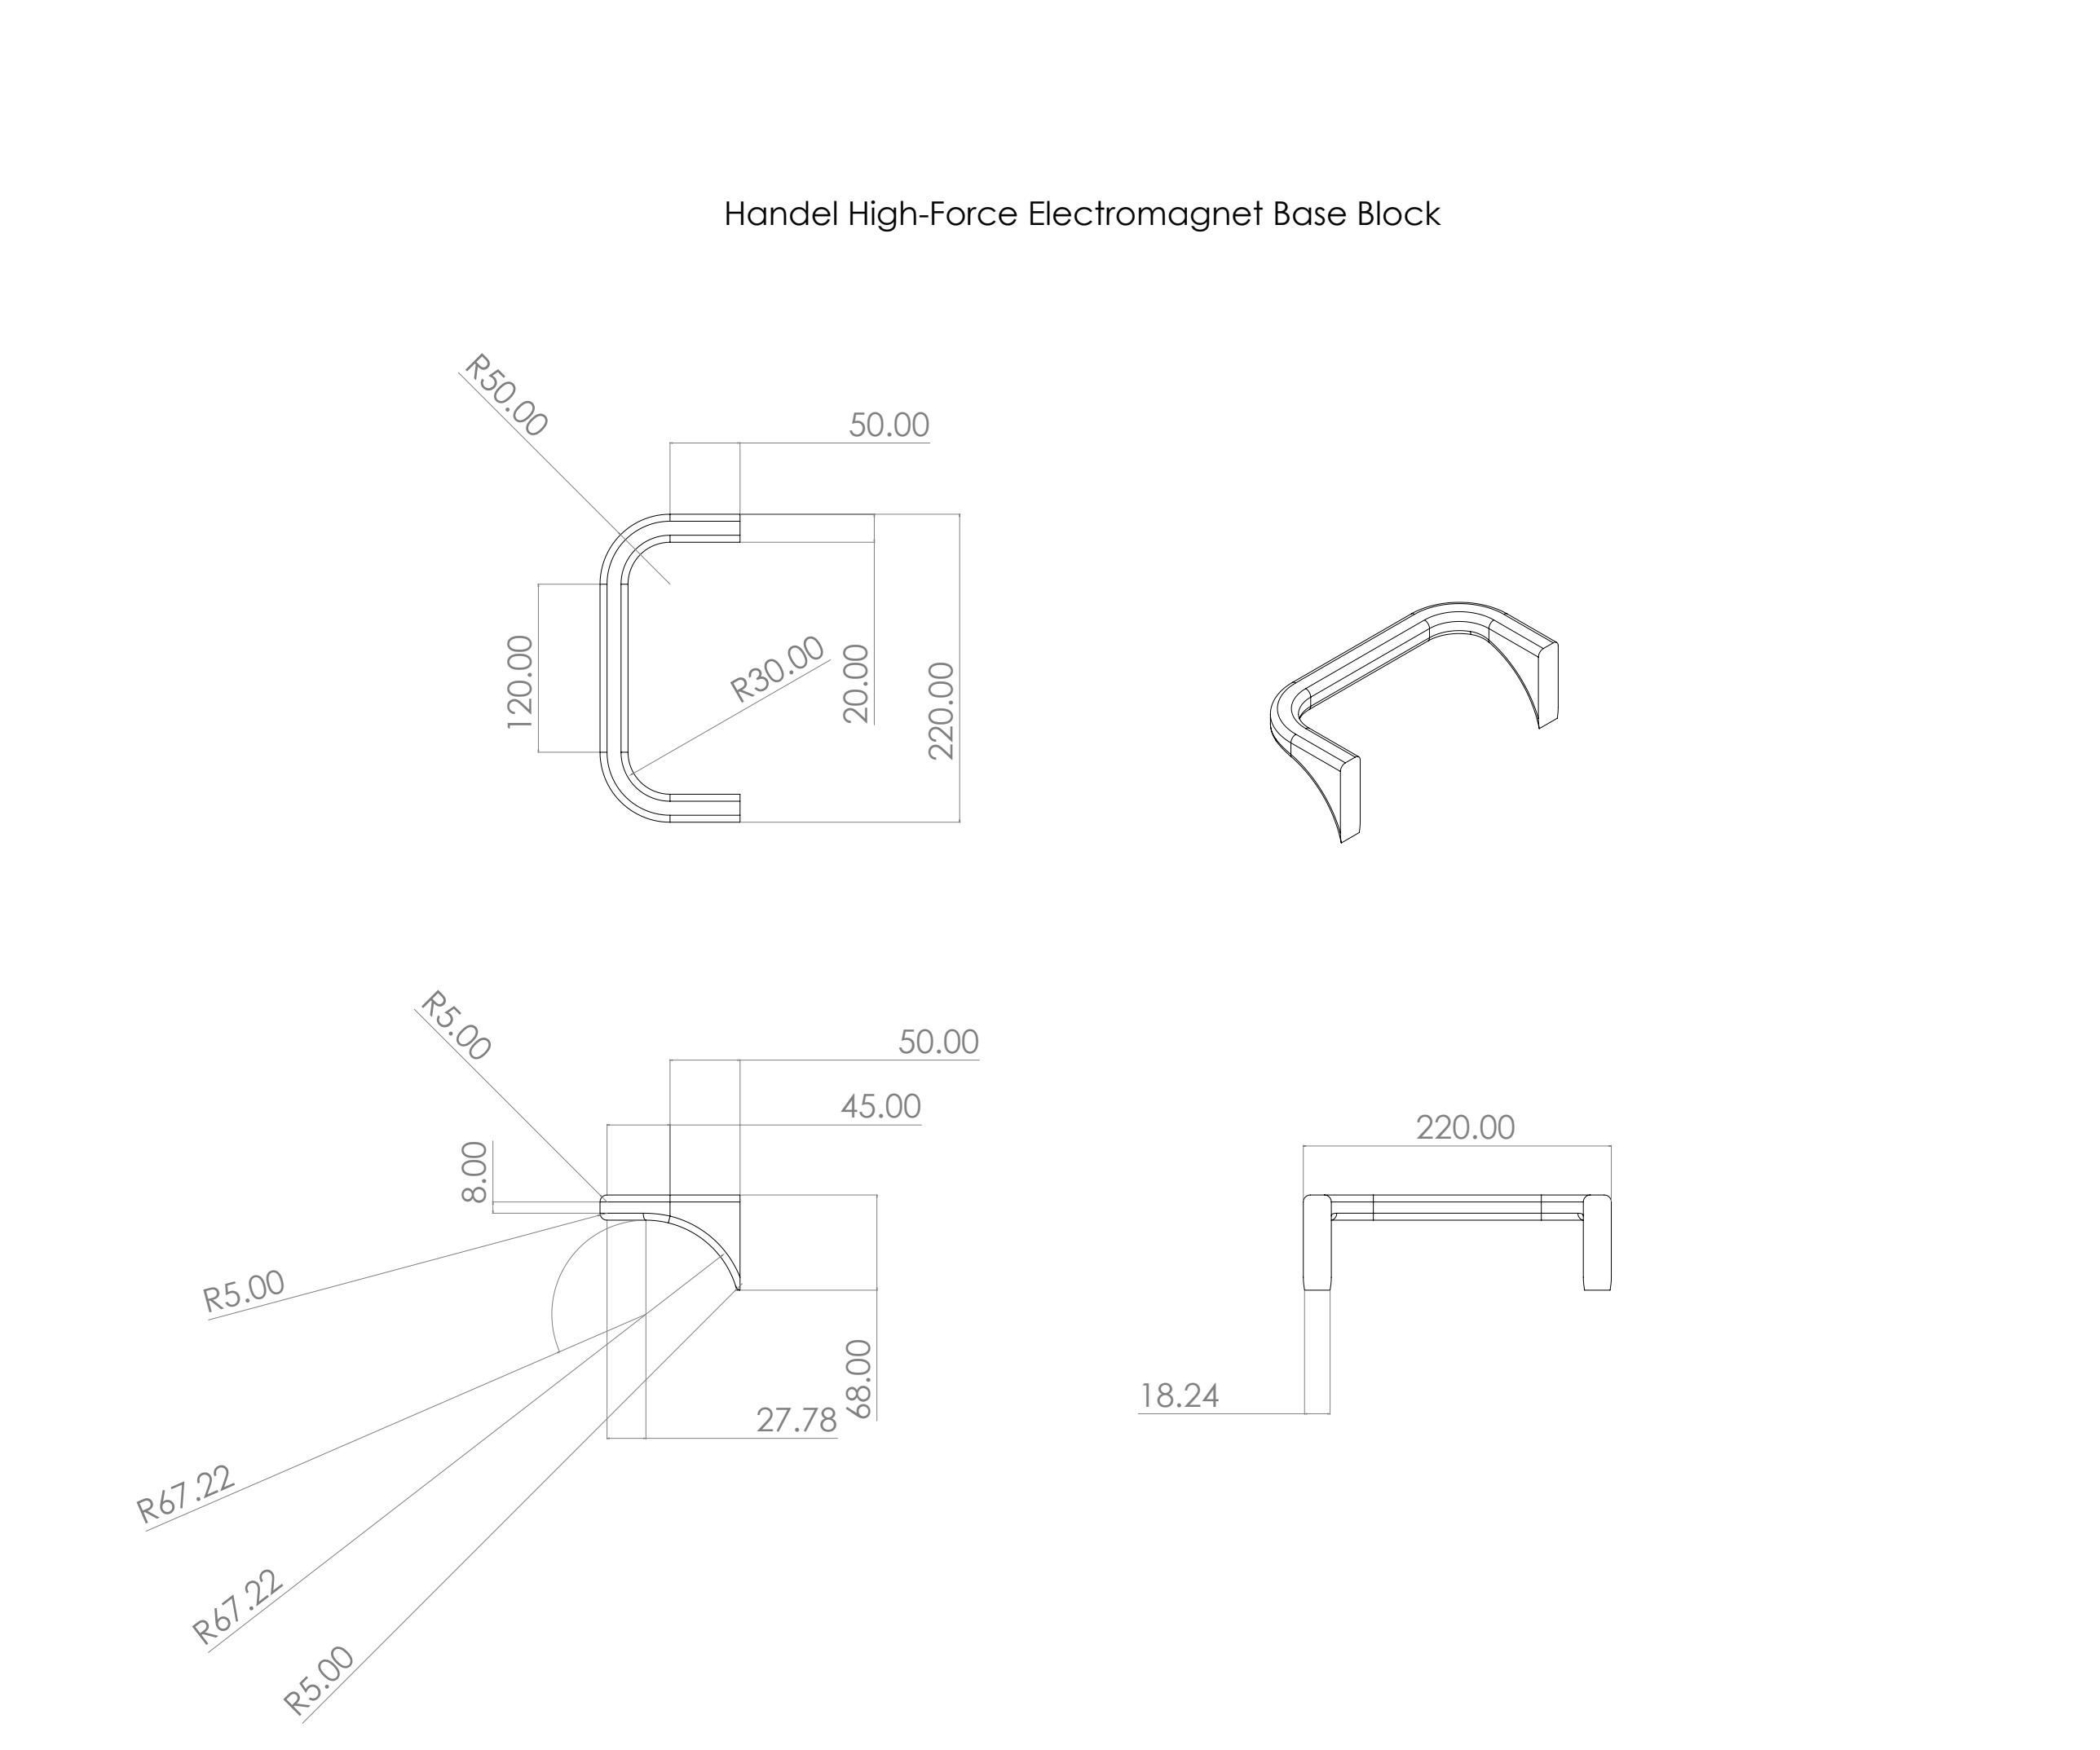
ISO-10303-21;
HEADER;
FILE_DESCRIPTION (('STEP AP214'),
    '1' );
FILE_NAME ('Handel High-Force Electromagnet Base Block.step',
    '2026-10-24T00:09:50',
    ( '' ),
    ( '' ),
    'SwSTEP 2.0',
    'SolidWorks 2025',
    '' );
FILE_SCHEMA (( 'AUTOMOTIVE_DESIGN' ));
ENDSEC;

DATA;
#89=CARTESIAN_POINT ( 'NONE',  ( -260.0000000000001137, -157.0000000000000284, -109.9999999999998721 ) ) ;
#164=CARTESIAN_POINT ( 'NONE',  ( -211.9382648910248861, -218.8137564101509724, 107.3933716542343575 ) ) ;
#173=ADVANCED_FACE ( 'NONE', ( #5707 ), #18920, .T. ) ;
#175=CYLINDRICAL_SURFACE ( 'NONE', #3295, 5.000000000000004441 ) ;
#187=DIRECTION ( 'NONE',  ( 0.000000000000000000, 0.000000000000000000, 1.000000000000000000 ) ) ;
#211=CARTESIAN_POINT ( 'NONE',  ( -260.0000000000001137, -220.0000000000000853, 110.0000000000000142 ) ) ;
#234=EDGE_LOOP ( 'NONE', ( #15831, #2366, #304, #19218 ) ) ;
#245=CARTESIAN_POINT ( 'NONE',  ( -260.0000000000001137, -165.0000000000001137, 60.00000000000002132 ) ) ;
#268=VERTEX_POINT ( 'NONE', #24222 ) ;
#275=VECTOR ( 'NONE', #1072, 1000.000000000000000 ) ;
#288=DIRECTION ( 'NONE',  ( -1.321694076934710155E-16, 1.000000000000000000, 0.000000000000000000 ) ) ;
#301=VERTEX_POINT ( 'NONE', #89 ) ;
#304=ORIENTED_EDGE ( 'NONE', *, *, #26732, .T. ) ;
#312=CARTESIAN_POINT ( 'NONE',  ( -213.1827219047386848, -216.7767438708612531, 105.0000000000000142 ) ) ;
#400=EDGE_CURVE ( 'NONE', #4420, #2951, #20623, .T. ) ;
#420=DIRECTION ( 'NONE',  ( 1.000000000000000000, 0.000000000000000000, 0.000000000000000000 ) ) ;
#473=ADVANCED_FACE ( 'NONE', ( #3894 ), #19413, .T. ) ;
#491=CARTESIAN_POINT ( 'NONE',  ( -270.0517793156885205, -165.1952670567707173, -88.29534001765418338 ) ) ;
#500=ORIENTED_EDGE ( 'NONE', *, *, #25165, .F. ) ;
#515=CARTESIAN_POINT ( 'NONE',  ( -263.9103269956589770, -171.2705086194569901, -104.9999999999999005 ) ) ;
#522=EDGE_LOOP ( 'NONE', ( #13816, #10578, #2122, #14859 ) ) ;
#539=ADVANCED_FACE ( 'NONE', ( #26156 ), #27734, .T. ) ;
#586=CARTESIAN_POINT ( 'NONE',  ( -210.0000000000000568, -157.0000000000000284, -94.99999999999987210 ) ) ;
#591=CARTESIAN_POINT ( 'NONE',  ( -260.0000000000001137, -167.0819201924624906, -109.9999999999998721 ) ) ;
#594=AXIS2_PLACEMENT_3D ( 'NONE', #26284, #2003, #28279 ) ;
#596=ORIENTED_EDGE ( 'NONE', *, *, #20943, .T. ) ;
#618=ORIENTED_EDGE ( 'NONE', *, *, #5223, .T. ) ;
#630=AXIS2_PLACEMENT_3D ( 'NONE', #3020, #873, #5034 ) ;
#631=LINE ( 'NONE', #7377, #27214 ) ;
#681=CARTESIAN_POINT ( 'NONE',  ( -262.5451564304015619, -171.6056065411685552, 105.0000000000519549 ) ) ;
#690=CARTESIAN_POINT ( 'NONE',  ( -210.0000000000000568, -210.8114316696540982, 110.0000000000000284 ) ) ;
#710=VECTOR ( 'NONE', #14587, 1000.000000000000000 ) ;
#721=AXIS2_PLACEMENT_3D ( 'NONE', #25156, #27436, #16685 ) ;
#750=VECTOR ( 'NONE', #15038, 1000.000000000000000 ) ;
#790=ORIENTED_EDGE ( 'NONE', *, *, #25750, .F. ) ;
#802=DIRECTION ( 'NONE',  ( 0.000000000000000000, 1.000000000000000000, 0.000000000000000000 ) ) ;
#817=CARTESIAN_POINT ( 'NONE',  ( -267.9882009536668193, -170.6226266830407496, 104.4279108778009828 ) ) ;
#821=DIRECTION ( 'NONE',  ( -0.8706753206611566043, -1.365180738000214426E-15, -0.4918581970360891842 ) ) ;
#844=CARTESIAN_POINT ( 'NONE',  ( -210.0000000000000000, -218.4793454996983826, 90.61920026979468901 ) ) ;
#865=CARTESIAN_POINT ( 'NONE',  ( -260.0000000000001137, -220.0000000000000853, 90.00000000000001421 ) ) ;
#873=DIRECTION ( 'NONE',  ( 0.9711705445023437466, -0.2383857661250380899, 0.000000000000000000 ) ) ;
#881=DIRECTION ( 'NONE',  ( -1.000000000000000000, 0.000000000000000000, 0.000000000000000000 ) ) ;
#921=DIRECTION ( 'NONE',  ( 4.540956701092242152E-16, 1.000000000000000000, 0.000000000000000000 ) ) ;
#932=CARTESIAN_POINT ( 'NONE',  ( -266.6125751775834942, -170.7865253013266056, -104.7181492081291765 ) ) ;
#973=CARTESIAN_POINT ( 'NONE',  ( -211.6502095576267948, -220.0000000000000568, -92.65159606798890479 ) ) ;
#974=TOROIDAL_SURFACE ( 'NONE', #19304, 44.99999999999999289, 5.000000000000000000 ) ;
#978=CARTESIAN_POINT ( 'NONE',  ( -295.0000000000001137, -170.0000000000001137, 60.00000000000002842 ) ) ;
#984=CARTESIAN_POINT ( 'NONE',  ( -260.0000000000001137, -157.0000000000000284, 60.00000000000002132 ) ) ;
#985=DIRECTION ( 'NONE',  ( -1.000000000000000000, 4.540956701092242152E-16, 0.000000000000000000 ) ) ;
#995=EDGE_LOOP ( 'NONE', ( #6255, #19786, #27111, #10655, #13692 ) ) ;
#1041=CYLINDRICAL_SURFACE ( 'NONE', #20624, 30.00000000000002842 ) ;
#1072=DIRECTION ( 'NONE',  ( -0.000000000000000000, -0.000000000000000000, -1.000000000000000000 ) ) ;
#1181=CARTESIAN_POINT ( 'NONE',  ( -210.0000000000000568, -210.8114316696540982, -89.99999999999987210 ) ) ;
#1212=CARTESIAN_POINT ( 'NONE',  ( -260.0000000000001137, -157.0000000000000284, 90.00000000000001421 ) ) ;
#1263=CARTESIAN_POINT ( 'NONE',  ( -266.7368518929977768, -170.8180696079899121, -94.49756868224339712 ) ) ;
#1264=LINE ( 'NONE', #16233, #14272 ) ;
#1292=LINE ( 'NONE', #27842, #24087 ) ;
#1329=CARTESIAN_POINT ( 'NONE',  ( -295.0000000000002274, -157.0000000000000284, -109.9999999999999858 ) ) ;
#1368=LINE ( 'NONE', #1645, #8748 ) ;
#1386=DIRECTION ( 'NONE',  ( -0.9711705445023439687, 0.2383857661250367854, 0.000000000000000000 ) ) ;
#1401=CARTESIAN_POINT ( 'NONE',  ( -262.3765419278357740, -171.6469950468170111, 89.94932042693801577 ) ) ;
#1411=CARTESIAN_POINT ( 'NONE',  ( -260.0000000000001137, -152.0000000000000284, 60.00000000000002132 ) ) ;
#1429=CARTESIAN_POINT ( 'NONE',  ( -279.1278187736259611, -165.0000000000001137, -106.1966075482097978 ) ) ;
#1432=AXIS2_PLACEMENT_3D ( 'NONE', #1964, #14773, #18933 ) ;
#1459=DIRECTION ( 'NONE',  ( 0.9239321509641974517, 1.061807240666843741E-15, 0.3825563754725196941 ) ) ;
#1468=PLANE ( 'NONE',  #18635 ) ;
#1469=DIRECTION ( 'NONE',  ( -1.321694076934710155E-16, 1.000000000000000000, 0.000000000000000000 ) ) ;
#1495=CARTESIAN_POINT ( 'NONE',  ( -210.0000000000000568, -220.0000000000000853, -109.1217062362807155 ) ) ;
#1508=DIRECTION ( 'NONE',  ( -1.321694076934710155E-16, 1.000000000000000000, 0.000000000000000000 ) ) ;
#1567=EDGE_LOOP ( 'NONE', ( #19464, #20883, #3429, #20222 ) ) ;
#1570=EDGE_CURVE ( 'NONE', #9462, #6741, #17622, .T. ) ;
#1583=TOROIDAL_SURFACE ( 'NONE', #22239, 45.00000000000000711, 5.000000000000000000 ) ;
#1590=EDGE_CURVE ( 'NONE', #16800, #27270, #27778, .T. ) ;
#1603=CIRCLE ( 'NONE', #25453, 5.000000000000004441 ) ;
#1620=EDGE_CURVE ( 'NONE', #28289, #17098, #27637, .T. ) ;
#1645=CARTESIAN_POINT ( 'NONE',  ( -210.0000000000000568, -220.0000000000000853, -89.99999999999987210 ) ) ;
#1655=CARTESIAN_POINT ( 'NONE',  ( -210.0000000000000568, -157.0000000000000284, 90.00000000000002842 ) ) ;
#1659=CYLINDRICAL_SURFACE ( 'NONE', #24420, 5.000000000000004441 ) ;
#1701=ORIENTED_EDGE ( 'NONE', *, *, #1570, .T. ) ;
#1715=CARTESIAN_POINT ( 'NONE',  ( -210.0000000000000568, -157.0000000000000284, 95.00000000000004263 ) ) ;
#1727=AXIS2_PLACEMENT_3D ( 'NONE', #17796, #18378, #985 ) ;
#1732=EDGE_LOOP ( 'NONE', ( #3173, #18800, #24385, #25189 ) ) ;
#1742=CYLINDRICAL_SURFACE ( 'NONE', #24674, 5.000000000000004441 ) ;
#1743=CARTESIAN_POINT ( 'NONE',  ( -260.0000000000001137, -152.0000000000000284, 105.0000000000000142 ) ) ;
#1762=DIRECTION ( 'NONE',  ( -1.321694076934710155E-16, 1.000000000000000000, 0.000000000000000000 ) ) ;
#1792=CARTESIAN_POINT ( 'NONE',  ( -262.5215738956072755, -166.3598102777078509, 89.99999999999998579 ) ) ;
#1810=ADVANCED_FACE ( 'NONE', ( #6661 ), #11116, .T. ) ;
#1812=PLANE ( 'NONE',  #12527 ) ;
#1817=CARTESIAN_POINT ( 'NONE',  ( -267.0129679999498649, -170.7675089197775264, -89.18277029719632765 ) ) ;
#1818=CARTESIAN_POINT ( 'NONE',  ( -266.3037744482016365, -165.6613878827935196, 89.35851331749265114 ) ) ;
#1821=CARTESIAN_POINT ( 'NONE',  ( -262.5802634612744555, -171.5969890882419406, -94.99999999999990052 ) ) ;
#1833=VECTOR ( 'NONE', #27757, 1000.000000000000000 ) ;
#1849=CARTESIAN_POINT ( 'NONE',  ( -271.2644327268766915, -165.3329768350718041, -108.7419004184296369 ) ) ;
#1882=EDGE_CURVE ( 'NONE', #21087, #5617, #8959, .T. ) ;
#1937=DIRECTION ( 'NONE',  ( 0.000000000000000000, 0.000000000000000000, -1.000000000000000000 ) ) ;
#1957=CARTESIAN_POINT ( 'NONE',  ( -266.0153270024459289, -170.9359483083451039, -94.62226971369513251 ) ) ;
#1958=CARTESIAN_POINT ( 'NONE',  ( -270.3796563303090466, -170.3242331377992684, 88.15587544550923838 ) ) ;
#1964=CARTESIAN_POINT ( 'NONE',  ( -277.2150368962633706, -237.2150368962634559, -109.9999999999998153 ) ) ;
#1993=ADVANCED_FACE ( 'NONE', ( #20301 ), #18155, .F. ) ;
#2002=CARTESIAN_POINT ( 'NONE',  ( -210.0000000000000568, -220.0000000000000853, 110.0000000000000284 ) ) ;
#2003=DIRECTION ( 'NONE',  ( -4.540956701092242152E-16, -1.000000000000000000, -0.000000000000000000 ) ) ;
#2019=EDGE_CURVE ( 'NONE', #17098, #12396, #27748, .T. ) ;
#2064=CARTESIAN_POINT ( 'NONE',  ( -262.5514013678064771, -171.6040736444017512, 105.0000000000000000 ) ) ;
#2073=ORIENTED_EDGE ( 'NONE', *, *, #6135, .T. ) ;
#2074=LINE ( 'NONE', #13160, #28386 ) ;
#2091=ORIENTED_EDGE ( 'NONE', *, *, #5972, .T. ) ;
#2096=CARTESIAN_POINT ( 'NONE',  ( -213.1248215185737820, -216.9499264940854744, 94.81074245358750829 ) ) ;
#2104=DIRECTION ( 'NONE',  ( -0.000000000000000000, -1.000000000000000000, -0.000000000000000000 ) ) ;
#2122=ORIENTED_EDGE ( 'NONE', *, *, #1590, .T. ) ;
#2143=DIRECTION ( 'NONE',  ( -1.000000000000000000, -9.204883169708156517E-49, 3.053113317719176542E-15 ) ) ;
#2151=SHAPE_DEFINITION_REPRESENTATION ( #25856, #3128 ) ;
#2258=AXIS2_PLACEMENT_3D ( 'NONE', #11059, #12938, #28277 ) ;
#2296=AXIS2_PLACEMENT_3D ( 'NONE', #27206, #12280, #10255 ) ;
#2320=DIRECTION ( 'NONE',  ( 0.000000000000000000, 0.000000000000000000, 1.000000000000000000 ) ) ;
#2351=CIRCLE ( 'NONE', #1432, 72.21503689626329958 ) ;
#2364=ORIENTED_EDGE ( 'NONE', *, *, #6001, .T. ) ;
#2366=ORIENTED_EDGE ( 'NONE', *, *, #15464, .T. ) ;
#2410=AXIS2_PLACEMENT_3D ( 'NONE', #19417, #16704, #20998 ) ;
#2419=CARTESIAN_POINT ( 'NONE',  ( -310.0000000000001137, -220.0000000000000853, -59.99999999999987210 ) ) ;
#2453=ADVANCED_FACE ( 'NONE', ( #8296 ), #5320, .T. ) ;
#2463=EDGE_LOOP ( 'NONE', ( #27973, #3663, #26251, #20729 ) ) ;
#2472=EDGE_CURVE ( 'NONE', #9488, #19744, #24227, .T. ) ;
#2494=ADVANCED_FACE ( 'NONE', ( #19915 ), #25006, .T. ) ;
#2502=DIRECTION ( 'NONE',  ( -1.321694076934710155E-16, 1.000000000000000000, 0.000000000000000000 ) ) ;
#2527=EDGE_CURVE ( 'NONE', #9488, #23090, #13611, .T. ) ;
#2532=LINE ( 'NONE', #22518, #11233 ) ;
#2542=ORIENTED_EDGE ( 'NONE', *, *, #24570, .T. ) ;
#2556=DIRECTION ( 'NONE',  ( -0.000000000000000000, -0.000000000000000000, 1.000000000000000000 ) ) ;
#2566=ADVANCED_FACE ( 'NONE', ( #24094 ), #8859, .T. ) ;
#2593=CARTESIAN_POINT ( 'NONE',  ( -213.1248215185737820, -216.9499264940855028, 105.1892575464125770 ) ) ;
#2608=DIRECTION ( 'NONE',  ( -1.000000000000000000, -0.000000000000000000, 2.775557561562887407E-16 ) ) ;
#2621=DIRECTION ( 'NONE',  ( -0.000000000000000000, -1.000000000000000000, -0.000000000000000000 ) ) ;
#2625=CARTESIAN_POINT ( 'NONE',  ( -260.0000000000001137, -170.0000000000001137, 60.00000000000002132 ) ) ;
#2634=ADVANCED_FACE ( 'NONE', ( #26951 ), #22652, .T. ) ;
#2676=CARTESIAN_POINT ( 'NONE',  ( -277.2150368962633706, -237.2150368962634559, 95.00000000000004263 ) ) ;
#2686=ORIENTED_EDGE ( 'NONE', *, *, #1570, .F. ) ;
#2687=DIRECTION ( 'NONE',  ( -0.000000000000000000, -0.000000000000000000, -1.000000000000000000 ) ) ;
#2715=STYLED_ITEM('',(#28420),#27732);
#2771=DIRECTION ( 'NONE',  ( 4.540956701092242152E-16, 1.000000000000000000, 0.000000000000000000 ) ) ;
#2777=CARTESIAN_POINT ( 'NONE',  ( -290.0000000000001137, -157.0000000000000284, 60.00000000000002842 ) ) ;
#2785=ORIENTED_EDGE ( 'NONE', *, *, #10230, .T. ) ;
#2798=CARTESIAN_POINT ( 'NONE',  ( -261.1919288306253293, -171.9377729149742038, -104.9999999999998721 ) ) ;
#2815=CARTESIAN_POINT ( 'NONE',  ( -272.9143904460767658, -165.1584295805091642, 108.4134862853730965 ) ) ;
#2830=B_SPLINE_CURVE_WITH_KNOTS ( 'NONE', 3,
 ( #15606, #24348, #4662, #13445, #19754, #4381, #12886, #22201, #19618, #26357, #24215, #23935 ),
 .UNSPECIFIED., .F., .F.,
 ( 4, 2, 2, 2, 2, 4 ),
 ( 0.000000000000000000, 0.004258726182425120153, 0.006388089273637603469, 0.008517452364850087651, 0.01277617854727505428, 0.01703490472970001918 ),
 .UNSPECIFIED. ) ;
#2857=CIRCLE ( 'NONE', #5602, 5.000000000000004441 ) ;
#2934=EDGE_CURVE ( 'NONE', #6860, #23545, #18607, .T. ) ;
#2945=CARTESIAN_POINT ( 'NONE',  ( -277.2150368962633706, -170.0000000000001137, 101.5769467933889558 ) ) ;
#2951=VERTEX_POINT ( 'NONE', #24194 ) ;
#2963=CARTESIAN_POINT ( 'NONE',  ( -261.1919288306253293, -171.9377729149742038, 105.0000000000000142 ) ) ;
#2972=DIRECTION ( 'NONE',  ( -1.321694076934710155E-16, 1.000000000000000000, 0.000000000000000000 ) ) ;
#2992=AXIS2_PLACEMENT_3D ( 'NONE', #7090, #26770, #20999 ) ;
#3020=CARTESIAN_POINT ( 'NONE',  ( -260.0000000000001137, -167.0819201924624906, 105.0000000000000142 ) ) ;
#3073=VECTOR ( 'NONE', #26874, 1000.000000000000000 ) ;
#3078=ORIENTED_EDGE ( 'NONE', *, *, #1620, .F. ) ;
#3095=CARTESIAN_POINT ( 'NONE',  ( -268.7660490202469532, -170.5116556248577524, 109.2537565056162379 ) ) ;
#3103=AXIS2_PLACEMENT_3D ( 'NONE', #28274, #8473, #17230 ) ;
#3128=SHAPE_REPRESENTATION ( 'Handel High-Force Electromagnet Base Block', ( #10637 ), #6979 ) ;
#3142=AXIS2_PLACEMENT_3D ( 'NONE', #11715, #22040, #15736 ) ;
#3144=DIRECTION ( 'NONE',  ( 0.000000000000000000, 0.000000000000000000, 1.000000000000000000 ) ) ;
#3147=VERTEX_POINT ( 'NONE', #2777 ) ;
#3173=ORIENTED_EDGE ( 'NONE', *, *, #15521, .T. ) ;
#3224=VERTEX_POINT ( 'NONE', #591 ) ;
#3236=CARTESIAN_POINT ( 'NONE',  ( -264.2078319525319898, -171.2518620402580325, 109.8556748947001296 ) ) ;
#3248=CARTESIAN_POINT ( 'NONE',  ( -260.0000000000001137, -167.0819201924624906, -94.99999999999987210 ) ) ;
#3272=DIRECTION ( 'NONE',  ( 0.3825563754725206378, 0.000000000000000000, 0.9239321509641971186 ) ) ;
#3295=AXIS2_PLACEMENT_3D ( 'NONE', #22146, #26589, #17410 ) ;
#3306=FACE_OUTER_BOUND ( 'NONE', #14305, .T. ) ;
#3316=PRODUCT_DEFINITION ( 'UNKNOWN', '', #4206, #7165 ) ;
#3325=CARTESIAN_POINT ( 'NONE',  ( -212.2419371577844345, -220.0000000000000853, -105.0000000000000284 ) ) ;
#3345=AXIS2_PLACEMENT_3D ( 'NONE', #5821, #12027, #12311 ) ;
#3349=AXIS2_PLACEMENT_3D ( 'NONE', #25379, #1386, #5699 ) ;
#3353=PLANE ( 'NONE',  #2296 ) ;
#3368=VERTEX_POINT ( 'NONE', #9476 ) ;
#3407=EDGE_CURVE ( 'NONE', #3147, #8779, #22883, .T. ) ;
#3418=CARTESIAN_POINT ( 'NONE',  ( -277.2150368962633706, -170.0000000000001137, -90.47363622314027509 ) ) ;
#3428=AXIS2_PLACEMENT_3D ( 'NONE', #27338, #9833, #11858 ) ;
#3429=ORIENTED_EDGE ( 'NONE', *, *, #9744, .F. ) ;
#3430=ORIENTED_EDGE ( 'NONE', *, *, #16149, .T. ) ;
#3448=FACE_OUTER_BOUND ( 'NONE', #16029, .T. ) ;
#3451=EDGE_CURVE ( 'NONE', #18918, #10091, #26206, .T. ) ;
#3457=CIRCLE ( 'NONE', #12242, 29.99999999999997158 ) ;
#3491=DIRECTION ( 'NONE',  ( -0.000000000000000000, -0.000000000000000000, 1.000000000000000000 ) ) ;
#3513=CARTESIAN_POINT ( 'NONE',  ( -210.0000000000000568, -216.9546086794800317, 109.5971846486504404 ) ) ;
#3520=DIRECTION ( 'NONE',  ( 1.000000000000000000, 0.000000000000000000, 2.775557561562887407E-16 ) ) ;
#3529=DIRECTION ( 'NONE',  ( 0.2383857661250380344, 0.9711705445023436356, 0.000000000000000000 ) ) ;
#3545=CARTESIAN_POINT ( 'NONE',  ( -277.2150368962633706, -170.0000000000001137, -90.47363622314027509 ) ) ;
#3547=CARTESIAN_POINT ( 'NONE',  ( -269.2495632547581863, -170.4544034111251278, 88.54864639839837537 ) ) ;
#3567=ORIENTED_EDGE ( 'NONE', *, *, #2527, .F. ) ;
#3577=CARTESIAN_POINT ( 'NONE',  ( -260.0000000000001137, -220.0000000000000853, 60.00000000000002132 ) ) ;
#3590=AXIS2_PLACEMENT_3D ( 'NONE', #15942, #20233, #420 ) ;
#3591=CARTESIAN_POINT ( 'NONE',  ( -266.4480630393687193, -165.8483660650564389, -109.6897131948989568 ) ) ;
#3602=CARTESIAN_POINT ( 'NONE',  ( -210.0000000000000568, -152.0000000000000284, -110.0000000000000284 ) ) ;
#3641=CARTESIAN_POINT ( 'NONE',  ( -210.0000000000000568, -210.8114316696540982, 90.00000000000002842 ) ) ;
#3663=ORIENTED_EDGE ( 'NONE', *, *, #5671, .F. ) ;
#3686=CARTESIAN_POINT ( 'NONE',  ( -266.9759726783797191, -165.5689182401532946, -89.18477089400076352 ) ) ;
#3699=DIRECTION ( 'NONE',  ( 0.000000000000000000, 0.000000000000000000, -1.000000000000000000 ) ) ;
#3702=VERTEX_POINT ( 'NONE', #14768 ) ;
#3720=CARTESIAN_POINT ( 'NONE',  ( -277.5942566850414437, -165.0000000000001705, -106.8315826960697450 ) ) ;
#3746=DIRECTION ( 'NONE',  ( -0.000000000000000000, -0.000000000000000000, 1.000000000000000000 ) ) ;
#3780=ORIENTED_EDGE ( 'NONE', *, *, #13513, .F. ) ;
#3781=AXIS2_PLACEMENT_3D ( 'NONE', #27138, #24992, #22976 ) ;
#3845=ORIENTED_EDGE ( 'NONE', *, *, #13749, .F. ) ;
#3873=LINE ( 'NONE', #12662, #17378 ) ;
#3884=ORIENTED_EDGE ( 'NONE', *, *, #1882, .F. ) ;
#3894=FACE_OUTER_BOUND ( 'NONE', #522, .T. ) ;
#3931=ADVANCED_FACE ( 'NONE', ( #21289 ), #14556, .T. ) ;
#3950=CARTESIAN_POINT ( 'NONE',  ( -260.0000000000001137, -167.0819201924624906, 90.00000000000001421 ) ) ;
#3969=DIRECTION ( 'NONE',  ( 1.321694076934710155E-16, -1.000000000000000000, 0.000000000000000000 ) ) ;
#3972=CARTESIAN_POINT ( 'NONE',  ( -268.8456629416622263, -165.3150191422601551, -88.69519881272435669 ) ) ;
#3973=CARTESIAN_POINT ( 'NONE',  ( -263.9427288773140390, -171.3087732700370225, 94.90640018636418063 ) ) ;
#3995=ADVANCED_FACE ( 'NONE', ( #12268 ), #1742, .T. ) ;
#4005=CARTESIAN_POINT ( 'NONE',  ( -305.0000000000001137, -165.0000000000000853, -59.99999999999987210 ) ) ;
#4017=CARTESIAN_POINT ( 'NONE',  ( -271.2500882473517549, -165.3342412936102050, -108.7452232840771558 ) ) ;
#4093=LINE ( 'NONE', #10997, #7349 ) ;
#4102=ORIENTED_EDGE ( 'NONE', *, *, #25165, .T. ) ;
#4115=CARTESIAN_POINT ( 'NONE',  ( -262.5702831125496459, -171.5994388877033998, -94.99999999999987210 ) ) ;
#4138=ORIENTED_EDGE ( 'NONE', *, *, #22755, .T. ) ;
#4161=CARTESIAN_POINT ( 'NONE',  ( -270.6159714707433182, -170.3110992094025278, -103.8707009556082994 ) ) ;
#4206=PRODUCT_DEFINITION_FORMATION_WITH_SPECIFIED_SOURCE ( 'ANY', '', #4537, .NOT_KNOWN. ) ;
#4251=VERTEX_POINT ( 'NONE', #14381 ) ;
#4255=CARTESIAN_POINT ( 'NONE',  ( -210.4359063544880541, -219.8547609215023328, 91.14353391724667119 ) ) ;
#4261=CARTESIAN_POINT ( 'NONE',  ( -210.0000000000000568, -152.0000000000000284, -110.0000000000000284 ) ) ;
#4264=CARTESIAN_POINT ( 'NONE',  ( -260.0000000000001137, -152.0000000000000284, -59.99999999999986500 ) ) ;
#4284=EDGE_LOOP ( 'NONE', ( #500, #10010, #26500, #14827 ) ) ;
#4381=CARTESIAN_POINT ( 'NONE',  ( -270.7820719900048516, -170.3051706208958365, 93.45761744549247396 ) ) ;
#4420=VERTEX_POINT ( 'NONE', #15232 ) ;
#4447=ORIENTED_EDGE ( 'NONE', *, *, #16149, .F. ) ;
#4503=ADVANCED_FACE ( 'NONE', ( #28133 ), #8757, .F. ) ;
#4519=CARTESIAN_POINT ( 'NONE',  ( -268.1249842685929821, -165.6674762674429076, 109.3623863443581570 ) ) ;
#4528=AXIS2_PLACEMENT_3D ( 'NONE', #22625, #921, #27062 ) ;
#4537=PRODUCT ( 'Handel High-Force Electromagnet Base Block', 'Handel High-Force Electromagnet Base Block', '', ( #21552 ) ) ;
#4544=FACE_OUTER_BOUND ( 'NONE', #11580, .T. ) ;
#4546=ADVANCED_FACE ( 'NONE', ( #13650 ), #25572, .T. ) ;
#4582=ORIENTED_EDGE ( 'NONE', *, *, #16178, .F. ) ;
#4593=ORIENTED_EDGE ( 'NONE', *, *, #25750, .T. ) ;
#4594=ADVANCED_FACE ( 'NONE', ( #11646 ), #26496, .T. ) ;
#4608=CARTESIAN_POINT ( 'NONE',  ( -210.0000000000000568, -220.0000000000000853, -89.99999999999987210 ) ) ;
#4611=CARTESIAN_POINT ( 'NONE',  ( -211.0655007229363207, -220.0000000000000568, -108.1818347287491378 ) ) ;
#4654=CARTESIAN_POINT ( 'NONE',  ( -295.0000000000001705, -152.0000000000000284, 60.00000000000002842 ) ) ;
#4658=CIRCLE ( 'NONE', #6486, 35.00000000000002842 ) ;
#4662=CARTESIAN_POINT ( 'NONE',  ( -274.7321073701114642, -170.0332518446063830, 91.86918944433702450 ) ) ;
#4680=CARTESIAN_POINT ( 'NONE',  ( -277.2150368962633706, -170.0000000000001137, -90.47363622314027509 ) ) ;
#4739=CARTESIAN_POINT ( 'NONE',  ( -295.0000000000001705, -165.0000000000001137, -59.99999999999986500 ) ) ;
#4757=DIRECTION ( 'NONE',  ( 1.000000000000000000, 0.000000000000000000, -2.775557561562887407E-16 ) ) ;
#4787=EDGE_LOOP ( 'NONE', ( #10218, #10585, #21921, #10657 ) ) ;
#4802=DIRECTION ( 'NONE',  ( 0.000000000000000000, 0.000000000000000000, -1.000000000000000000 ) ) ;
#4823=DIRECTION ( 'NONE',  ( -1.000000000000000000, 0.000000000000000000, 0.000000000000000000 ) ) ;
#4852=UNCERTAINTY_MEASURE_WITH_UNIT (LENGTH_MEASURE( 1.000000000000000082E-05 ), #24383, 'distance_accuracy_value', 'NONE');
#5022=ORIENTED_EDGE ( 'NONE', *, *, #5982, .T. ) ;
#5032=EDGE_CURVE ( 'NONE', #5806, #16800, #18347, .T. ) ;
#5034=DIRECTION ( 'NONE',  ( 0.2383857661250380344, 0.9711705445023436356, 0.000000000000000000 ) ) ;
#5051=ORIENTED_EDGE ( 'NONE', *, *, #6001, .F. ) ;
#5074=CARTESIAN_POINT ( 'NONE',  ( -262.5249090614869374, -166.4079007703013247, -89.92078834904907580 ) ) ;
#5116=CARTESIAN_POINT ( 'NONE',  ( -279.1278187736259611, -170.0000000000001421, 106.1966075482099683 ) ) ;
#5132=ORIENTED_EDGE ( 'NONE', *, *, #28205, .F. ) ;
#5146=EDGE_CURVE ( 'NONE', #16800, #12640, #24714, .T. ) ;
#5157=AXIS2_PLACEMENT_3D ( 'NONE', #15697, #10951, #13397 ) ;
#5223=EDGE_CURVE ( 'NONE', #18214, #19744, #5687, .T. ) ;
#5257=DIRECTION ( 'NONE',  ( -1.000000000000000000, 0.000000000000000000, -0.000000000000000000 ) ) ;
#5279=ORIENTED_EDGE ( 'NONE', *, *, #10174, .T. ) ;
#5295=DIRECTION ( 'NONE',  ( -0.000000000000000000, -0.000000000000000000, 1.000000000000000000 ) ) ;
#5305=ORIENTED_EDGE ( 'NONE', *, *, #22027, .F. ) ;
#5320=( BOUNDED_SURFACE ( )  B_SPLINE_SURFACE ( 3, 2, ( 
 ( #25811, #14913, #28097 ),
 ( #5714, #1401, #23667 ),
 ( #3973, #12760, #6276 ),
 ( #21500, #15050, #19495 ),
 ( #17332, #12340, #1818 ),
 ( #10173, #10592, #28239 ),
 ( #19348, #3547, #12901 ),
 ( #21648, #1958, #14488 ),
 ( #23245, #16779, #18930 ),
 ( #27673, #8013, #13463 ),
 ( #11459, #15195, #15482 ),
 ( #9003, #23952, #22072 ) ),
 .UNSPECIFIED., .F., .F., .F. ) 
 B_SPLINE_SURFACE_WITH_KNOTS ( ( 4, 2, 2, 2, 2, 4 ),
 ( 3, 3 ),
 ( 0.000000000000000000, 0.004509302159734392135, 0.009018604319468784269, 0.01127325539933598034, 0.01352790647920317640, 0.01803720863893756854 ),
 ( 0.000000000000000000, 1.000000000000000000 ),
 .UNSPECIFIED. ) 
 GEOMETRIC_REPRESENTATION_ITEM ( )  RATIONAL_B_SPLINE_SURFACE ( (
 ( 1.000000000000000000, 0.7071067811865475727, 1.000000000000000000),
 ( 1.000000000000000000, 0.7035406144708270526, 1.000000000000000000),
 ( 1.000000000000000000, 0.7008848705186870864, 1.000000000000000000),
 ( 1.000000000000000000, 0.6974083274405008526, 1.000000000000000000),
 ( 1.000000000000000000, 0.6965884901777600335, 1.000000000000000000),
 ( 1.000000000000000000, 0.6967133934288484154, 1.000000000000000000),
 ( 1.000000000000000000, 0.6969819717335956621, 1.000000000000000000),
 ( 1.000000000000000000, 0.6979534373899805022, 1.000000000000000000),
 ( 1.000000000000000000, 0.6986531993633946502, 1.000000000000000000),
 ( 1.000000000000000000, 0.7013382012354564266, 1.000000000000000000),
 ( 1.000000000000000000, 0.7039093929050953546, 1.000000000000000000),
 ( 1.000000000000000000, 0.7071067811865475727, 1.000000000000000000) ) ) 
 REPRESENTATION_ITEM ( '' )  SURFACE ( )  );
#5365=LINE ( 'NONE', #13723, #16606 ) ;
#5377=AXIS2_PLACEMENT_3D ( 'NONE', #3602, #5484, #20857 ) ;
#5382=ORIENTED_EDGE ( 'NONE', *, *, #12688, .F. ) ;
#5387=CARTESIAN_POINT ( 'NONE',  ( -212.2419371577844345, -220.0000000000000853, -94.99999999999987210 ) ) ;
#5477=EDGE_CURVE ( 'NONE', #10903, #10018, #16476, .T. ) ;
#5484=DIRECTION ( 'NONE',  ( 0.000000000000000000, -1.000000000000000000, -0.000000000000000000 ) ) ;
#5499=CARTESIAN_POINT ( 'NONE',  ( -272.4438906011233712, -165.0368527442270477, -87.32790004433633158 ) ) ;
#5507=ORIENTED_EDGE ( 'NONE', *, *, #1882, .T. ) ;
#5526=CARTESIAN_POINT ( 'NONE',  ( -210.0000000000000568, -210.8114316696540982, -110.0000000000000284 ) ) ;
#5534=CARTESIAN_POINT ( 'NONE',  ( -210.0000000000000000, -212.3568517473289035, 110.0000000000000000 ) ) ;
#5541=CARTESIAN_POINT ( 'NONE',  ( -267.2505360800719814, -170.7220645054522663, 109.5009084174815541 ) ) ;
#5553=FACE_OUTER_BOUND ( 'NONE', #10103, .T. ) ;
#5554=VERTEX_POINT ( 'NONE', #21544 ) ;
#5555=CARTESIAN_POINT ( 'NONE',  ( -279.1278187736259611, -165.0000000000001137, -106.1966075482097978 ) ) ;
#5564=CARTESIAN_POINT ( 'NONE',  ( -290.0000000000001705, -157.0000000000000284, -59.99999999999986500 ) ) ;
#5602=AXIS2_PLACEMENT_3D ( 'NONE', #20556, #7498, #881 ) ;
#5617=VERTEX_POINT ( 'NONE', #7393 ) ;
#5662=ORIENTED_EDGE ( 'NONE', *, *, #5477, .T. ) ;
#5669=CARTESIAN_POINT ( 'NONE',  ( -210.0000000000000853, -216.9546086794800601, -109.5971846486504830 ) ) ;
#5671=EDGE_CURVE ( 'NONE', #23545, #15321, #3873, .T. ) ;
#5687=LINE ( 'NONE', #23213, #11873 ) ;
#5699=DIRECTION ( 'NONE',  ( -0.2383857661250380344, -0.9711705445023436356, 0.000000000000000000 ) ) ;
#5707=FACE_OUTER_BOUND ( 'NONE', #995, .T. ) ;
#5712=CARTESIAN_POINT ( 'NONE',  ( -266.7040755562055097, -170.8232809441065001, -94.50355751542548433 ) ) ;
#5714=CARTESIAN_POINT ( 'NONE',  ( -262.5700334248197123, -171.5995001766305847, 94.99999999990480148 ) ) ;
#5723=ORIENTED_EDGE ( 'NONE', *, *, #19780, .F. ) ;
#5728=ORIENTED_EDGE ( 'NONE', *, *, #27879, .T. ) ;
#5748=EDGE_CURVE ( 'NONE', #22565, #22186, #7330, .T. ) ;
#5775=ADVANCED_FACE ( 'NONE', ( #10778 ), #23374, .T. ) ;
#5798=ORIENTED_EDGE ( 'NONE', *, *, #25915, .T. ) ;
#5806=VERTEX_POINT ( 'NONE', #27132 ) ;
#5820=CARTESIAN_POINT ( 'NONE',  ( -260.0000000000001137, -165.0000000000001137, -59.99999999999986500 ) ) ;
#5821=CARTESIAN_POINT ( 'NONE',  ( -310.0000000000001137, -220.0000000000000853, -59.99999999999987210 ) ) ;
#5832=DIRECTION ( 'NONE',  ( -1.000000000000000000, 0.000000000000000000, 0.000000000000000000 ) ) ;
#5842=VERTEX_POINT ( 'NONE', #26990 ) ;
#5847=CARTESIAN_POINT ( 'NONE',  ( -212.1902656986470390, -220.0000000000000284, -94.18570773969327092 ) ) ;
#5849=CARTESIAN_POINT ( 'NONE',  ( -273.6179505379467400, -164.9999999998308624, -86.76301814019983283 ) ) ;
#5875=B_SPLINE_CURVE_WITH_KNOTS ( 'NONE', 3,
 ( #3950, #1792, #10569, #19325, #15317, #26349, #15028, #23780, #17449, #21621 ),
 .UNSPECIFIED., .F., .F.,
 ( 4, 2, 2, 2, 4 ),
 ( 0.000000000000000000, 0.007751866621267358357, 0.009689833276584160215, 0.01162779993190096207, 0.01550373324253456232 ),
 .UNSPECIFIED. ) ;
#5881=DIRECTION ( 'NONE',  ( 0.000000000000000000, 0.000000000000000000, 1.000000000000000000 ) ) ;
#5894=CARTESIAN_POINT ( 'NONE',  ( -271.9547679543769618, -170.1928761609053993, -103.5145866598865183 ) ) ;
#5936=CARTESIAN_POINT ( 'NONE',  ( -295.0000000000002274, -152.0000000000000284, -59.99999999999986500 ) ) ;
#5937=AXIS2_PLACEMENT_3D ( 'NONE', #20996, #1459, #10234 ) ;
#5969=DIRECTION ( 'NONE',  ( -2.775557561562887407E-16, -3.668437989309015850E-32, 1.000000000000000000 ) ) ;
#5971=ORIENTED_EDGE ( 'NONE', *, *, #20762, .T. ) ;
#5972=EDGE_CURVE ( 'NONE', #6357, #18214, #20609, .T. ) ;
#5982=EDGE_CURVE ( 'NONE', #24757, #12396, #14205, .T. ) ;
#5990=CARTESIAN_POINT ( 'NONE',  ( -262.3767685073270286, -171.6469394300385432, -89.94931073348448081 ) ) ;
#6001=EDGE_CURVE ( 'NONE', #21738, #15321, #6003, .T. ) ;
#6002=TOROIDAL_SURFACE ( 'NONE', #16113, 72.21503689626331379, 5.000000000000000000 ) ;
#6003=LINE ( 'NONE', #10181, #17854 ) ;
#6039=CARTESIAN_POINT ( 'NONE',  ( -273.2081292221210447, -170.0913695707084514, -108.2505382271841086 ) ) ;
#6070=VERTEX_POINT ( 'NONE', #3418 ) ;
#6077=CARTESIAN_POINT ( 'NONE',  ( -295.0000000000001705, -170.0000000000001137, -59.99999999999986500 ) ) ;
#6114=DIRECTION ( 'NONE',  ( -1.321694076934710155E-16, 1.000000000000000000, 0.000000000000000000 ) ) ;
#6115=DIRECTION ( 'NONE',  ( -1.000000000000000000, 4.540956701092242152E-16, 0.000000000000000000 ) ) ;
#6116=LINE ( 'NONE', #14746, #23778 ) ;
#6132=CARTESIAN_POINT ( 'NONE',  ( -211.4917091876254744, -219.2061850725015120, 92.08741365143876578 ) ) ;
#6135=EDGE_CURVE ( 'NONE', #12640, #6070, #12377, .T. ) ;
#6136=CARTESIAN_POINT ( 'NONE',  ( -274.7557459110828972, -170.0000000000001137, -86.12025961983449918 ) ) ;
#6175=DIRECTION ( 'NONE',  ( 1.000000000000000000, 0.000000000000000000, -2.775557561562887407E-16 ) ) ;
#6255=ORIENTED_EDGE ( 'NONE', *, *, #12010, .T. ) ;
#6276=CARTESIAN_POINT ( 'NONE',  ( -262.5332230410764396, -166.4061304486595532, 89.91977158827830863 ) ) ;
#6323=EDGE_CURVE ( 'NONE', #27440, #5617, #23847, .T. ) ;
#6336=LINE ( 'NONE', #27739, #13471 ) ;
#6343=ORIENTED_EDGE ( 'NONE', *, *, #25057, .T. ) ;
#6357=VERTEX_POINT ( 'NONE', #24815 ) ;
#6373=AXIS2_PLACEMENT_3D ( 'NONE', #25580, #3746, #15114 ) ;
#6414=CARTESIAN_POINT ( 'NONE',  ( -212.5524510162168212, -218.0941723687616900, 93.50253975917524940 ) ) ;
#6486=AXIS2_PLACEMENT_3D ( 'NONE', #19894, #19327, #10857 ) ;
#6496=CARTESIAN_POINT ( 'NONE',  ( -211.8239278721113408, -220.0000000000001421, -106.9797831932409622 ) ) ;
#6502=EDGE_CURVE ( 'NONE', #5842, #6860, #4093, .T. ) ;
#6516=CARTESIAN_POINT ( 'NONE',  ( -210.0000000000000568, -220.0000000000000853, 110.0000000000000284 ) ) ;
#6550=EDGE_LOOP ( 'NONE', ( #5728, #7123, #5723, #27554 ) ) ;
#6555=CARTESIAN_POINT ( 'NONE',  ( -274.7557459110829541, -165.0000000000001421, 86.12025961983462707 ) ) ;
#6557=CIRCLE ( 'NONE', #9314, 4.999999999999992895 ) ;
#6567=EDGE_CURVE ( 'NONE', #17968, #27440, #5875, .T. ) ;
#6581=( NAMED_UNIT ( * ) SI_UNIT ( $, .STERADIAN. ) SOLID_ANGLE_UNIT ( ) );
#6640=CARTESIAN_POINT ( 'NONE',  ( -210.6511289989136912, -220.0000000000000568, -108.6306965739821067 ) ) ;
#6661=FACE_OUTER_BOUND ( 'NONE', #13997, .T. ) ;
#6666=CARTESIAN_POINT ( 'NONE',  ( -272.0365926943243835, -170.1453898595840144, 103.5646192279123170 ) ) ;
#6722=ORIENTED_EDGE ( 'NONE', *, *, #27605, .F. ) ;
#6731=EDGE_CURVE ( 'NONE', #13530, #21087, #8096, .T. ) ;
#6736=FACE_OUTER_BOUND ( 'NONE', #22344, .T. ) ;
#6741=VERTEX_POINT ( 'NONE', #25192 ) ;
#6775=CARTESIAN_POINT ( 'NONE',  ( -210.0000000000000568, -157.0000000000000284, 90.00000000000002842 ) ) ;
#6814=ORIENTED_EDGE ( 'NONE', *, *, #19780, .T. ) ;
#6818=ADVANCED_FACE ( 'NONE', ( #23185 ), #3353, .T. ) ;
#6823=CARTESIAN_POINT ( 'NONE',  ( -272.9248965604650721, -165.1577306887913892, 108.4106317744307262 ) ) ;
#6860=VERTEX_POINT ( 'NONE', #25893 ) ;
#6927=CARTESIAN_POINT ( 'NONE',  ( -295.0000000000001705, -157.0000000000000284, -59.99999999999986500 ) ) ;
#6938=DIRECTION ( 'NONE',  ( -1.000000000000000000, 7.930164461608265370E-16, 0.000000000000000000 ) ) ;
#6965=CARTESIAN_POINT ( 'NONE',  ( -274.6324364865060943, -170.0364449491623589, -102.6462360633263984 ) ) ;
#6979=( GEOMETRIC_REPRESENTATION_CONTEXT ( 3 ) GLOBAL_UNCERTAINTY_ASSIGNED_CONTEXT ( ( #13789 ) ) GLOBAL_UNIT_ASSIGNED_CONTEXT ( ( #15284, #8380, #22012 ) ) REPRESENTATION_CONTEXT ( 'NONE', 'WORKASPACE' ) );
#6983=LINE ( 'NONE', #17471, #9183 ) ;
#7000=CARTESIAN_POINT ( 'NONE',  ( -210.0000000000000568, -152.0000000000000284, 95.00000000000004263 ) ) ;
#7023=ADVANCED_FACE ( 'NONE', ( #25281 ), #25139, .F. ) ;
#7030=CIRCLE ( 'NONE', #3349, 4.999999999999992895 ) ;
#7090=CARTESIAN_POINT ( 'NONE',  ( -260.0000000000001137, -170.0000000000001137, -59.99999999999986500 ) ) ;
#7123=ORIENTED_EDGE ( 'NONE', *, *, #24060, .F. ) ;
#7138=DIRECTION ( 'NONE',  ( -4.625929269271489858E-16, 2.100614451407711032E-31, -1.000000000000000000 ) ) ;
#7146=ORIENTED_EDGE ( 'NONE', *, *, #9496, .T. ) ;
#7165=PRODUCT_DEFINITION_CONTEXT ( 'detailed design', #24702, 'design' ) ;
#7293=ADVANCED_FACE ( 'NONE', ( #4544 ), #6002, .T. ) ;
#7324=( GEOMETRIC_REPRESENTATION_CONTEXT ( 3 ) GLOBAL_UNCERTAINTY_ASSIGNED_CONTEXT ( ( #4852 ) ) GLOBAL_UNIT_ASSIGNED_CONTEXT ( ( #24383, #17774, #6581 ) ) REPRESENTATION_CONTEXT ( 'NONE', 'WORKASPACE' ) );
#7326=DIRECTION ( 'NONE',  ( 0.000000000000000000, 0.000000000000000000, -1.000000000000000000 ) ) ;
#7330=CIRCLE ( 'NONE', #2258, 45.00000000000000711 ) ;
#7347=( BOUNDED_SURFACE ( )  B_SPLINE_SURFACE ( 3, 2, ( 
 ( #8628, #25567, #8342 ),
 ( #28286, #17101, #17381 ),
 ( #28145, #17240, #3591 ),
 ( #4161, #25998, #4017 ),
 ( #5894, #6039, #12947 ),
 ( #21550, #10499, #21266 ),
 ( #26143, #12386, #15100 ),
 ( #23857, #14667, #21122 ) ),
 .UNSPECIFIED., .F., .F., .F. ) 
 B_SPLINE_SURFACE_WITH_KNOTS ( ( 4, 2, 2, 4 ),
 ( 3, 3 ),
 ( 1.734723475976807094E-18, 0.008853360896355882970, 0.01328004134453382445, 0.01770672179271176594 ),
 ( 0.000000000000000000, 1.000000000000000000 ),
 .UNSPECIFIED. ) 
 GEOMETRIC_REPRESENTATION_ITEM ( )  RATIONAL_B_SPLINE_SURFACE ( (
 ( 1.000000000000000000, 0.7071067811865475727, 1.000000000000000000),
 ( 1.000000000000000000, 0.7125463296805260027, 1.000000000000000000),
 ( 1.000000000000000000, 0.7151690839163242774, 1.000000000000000000),
 ( 1.000000000000000000, 0.7150975281021120233, 1.000000000000000000),
 ( 1.000000000000000000, 0.7144031600608887755, 1.000000000000000000),
 ( 1.000000000000000000, 0.7116947786415229737, 1.000000000000000000),
 ( 1.000000000000000000, 0.7096971281777894047, 1.000000000000000000),
 ( 1.000000000000000000, 0.7071067811865465735, 1.000000000000000000) ) ) 
 REPRESENTATION_ITEM ( '' )  SURFACE ( )  );
#7349=VECTOR ( 'NONE', #6114, 1000.000000000000000 ) ;
#7377=CARTESIAN_POINT ( 'NONE',  ( -210.0000000000000568, -220.0000000000000853, 110.0000000000000284 ) ) ;
#7393=CARTESIAN_POINT ( 'NONE',  ( -277.2150368962633706, -170.0000000000001137, 90.47363622314043141 ) ) ;
#7402=EDGE_LOOP ( 'NONE', ( #16309, #22052, #7967, #596 ) ) ;
#7404=ORIENTED_EDGE ( 'NONE', *, *, #27605, .T. ) ;
#7427=FACE_OUTER_BOUND ( 'NONE', #234, .T. ) ;
#7445=ORIENTED_EDGE ( 'NONE', *, *, #12688, .T. ) ;
#7457=CARTESIAN_POINT ( 'NONE',  ( -210.0000000000000853, -216.9546086794800317, 90.40281535134961644 ) ) ;
#7476=ORIENTED_EDGE ( 'NONE', *, *, #25409, .F. ) ;
#7490=CIRCLE ( 'NONE', #23537, 5.000000000000004441 ) ;
#7498=DIRECTION ( 'NONE',  ( 0.000000000000000000, 0.000000000000000000, -1.000000000000000000 ) ) ;
#7558=EDGE_LOOP ( 'NONE', ( #26937, #19974, #4102, #19024, #21588, #15542, #2364, #5798 ) ) ;
#7593=CARTESIAN_POINT ( 'NONE',  ( -211.9731542214773583, -220.0000000000000853, -93.39625318057545655 ) ) ;
#7728=CARTESIAN_POINT ( 'NONE',  ( -212.2419371577845197, -220.0000000000000568, -94.58889440303579477 ) ) ;
#7731=CARTESIAN_POINT ( 'NONE',  ( -260.0000000000001137, -157.0000000000000284, -59.99999999999986500 ) ) ;
#7738=FACE_OUTER_BOUND ( 'NONE', #4787, .T. ) ;
#7746=ORIENTED_EDGE ( 'NONE', *, *, #2527, .T. ) ;
#7849=TOROIDAL_SURFACE ( 'NONE', #11542, 72.21503689626331379, 5.000000000000000000 ) ;
#7861=CARTESIAN_POINT ( 'NONE',  ( -212.0372611395816875, -220.0000000000000568, -93.59249812946184477 ) ) ;
#7899=AXIS2_PLACEMENT_3D ( 'NONE', #27570, #27712, #7909 ) ;
#7900=CARTESIAN_POINT ( 'NONE',  ( -272.8608663272381136, -165.2063914494869721, -108.3460931901318673 ) ) ;
#7909=DIRECTION ( 'NONE',  ( 1.000000000000000000, 3.004539147878382249E-48, -2.775557561562887407E-16 ) ) ;
#7921=DIRECTION ( 'NONE',  ( -1.000000000000000000, 0.000000000000000000, -1.850371707708595943E-15 ) ) ;
#7926=VECTOR ( 'NONE', #2502, 1000.000000000000000 ) ;
#7933=ADVANCED_FACE ( 'NONE', ( #17234 ), #7849, .T. ) ;
#7958=CARTESIAN_POINT ( 'NONE',  ( -310.0000000000001137, -165.0000000000001137, -59.99999999999987210 ) ) ;
#7967=ORIENTED_EDGE ( 'NONE', *, *, #17860, .T. ) ;
#7968=VECTOR ( 'NONE', #2608, 1000.000000000000000 ) ;
#7973=EDGE_CURVE ( 'NONE', #9462, #13525, #8189, .T. ) ;
#7990=CYLINDRICAL_SURFACE ( 'NONE', #19655, 5.000000000000004441 ) ;
#8006=CARTESIAN_POINT ( 'NONE',  ( -260.0000000000001137, -220.0000000000000853, 60.00000000000002132 ) ) ;
#8013=CARTESIAN_POINT ( 'NONE',  ( -272.5977457686555567, -170.1167710987052146, 87.25339983416321843 ) ) ;
#8025=CIRCLE ( 'NONE', #20855, 5.000000000000004441 ) ;
#8031=CIRCLE ( 'NONE', #27738, 67.21503689626328537 ) ;
#8051=ORIENTED_EDGE ( 'NONE', *, *, #13749, .T. ) ;
#8065=DIRECTION ( 'NONE',  ( -4.540956701092242152E-16, -1.000000000000000000, -0.000000000000000000 ) ) ;
#8075=DIRECTION ( 'NONE',  ( -0.000000000000000000, -0.000000000000000000, 1.000000000000000000 ) ) ;
#8096=LINE ( 'NONE', #20738, #1833 ) ;
#8097=CARTESIAN_POINT ( 'NONE',  ( -305.0000000000001137, -165.0000000000001137, 60.00000000000002842 ) ) ;
#8147=CARTESIAN_POINT ( 'NONE',  ( -210.8169819562698137, -219.6631312228495574, 91.44098042302121598 ) ) ;
#8189=LINE ( 'NONE', #2002, #15654 ) ;
#8210=AXIS2_PLACEMENT_3D ( 'NONE', #24452, #11096, #8939 ) ;
#8218=AXIS2_PLACEMENT_3D ( 'NONE', #21232, #27541, #3272 ) ;
#8232=CARTESIAN_POINT ( 'NONE',  ( -277.2150368962633706, -237.2150368962634559, 90.00000000000002842 ) ) ;
#8282=ORIENTED_EDGE ( 'NONE', *, *, #6502, .T. ) ;
#8296=FACE_OUTER_BOUND ( 'NONE', #13170, .T. ) ;
#8311=ORIENTED_EDGE ( 'NONE', *, *, #10230, .F. ) ;
#8342=CARTESIAN_POINT ( 'NONE',  ( -260.0000000000001137, -167.0819201924624906, -109.9999999999998721 ) ) ;
#8380=( NAMED_UNIT ( * ) PLANE_ANGLE_UNIT ( ) SI_UNIT ( $, .RADIAN. ) );
#8384=ORIENTED_EDGE ( 'NONE', *, *, #28205, .T. ) ;
#8440=CARTESIAN_POINT ( 'NONE',  ( -262.5386721175036655, -166.4045974903192473, -89.91974897482165829 ) ) ;
#8473=DIRECTION ( 'NONE',  ( -0.000000000000000000, -0.000000000000000000, 1.000000000000000000 ) ) ;
#8513=AXIS2_PLACEMENT_3D ( 'NONE', #2625, #2771, #6938 ) ;
#8547=CARTESIAN_POINT ( 'NONE',  ( -260.0000000000001137, -167.0819201924624906, 90.00000000000001421 ) ) ;
#8566=CARTESIAN_POINT ( 'NONE',  ( -261.6207973860045968, -166.7238599877898935, 110.0000000000000142 ) ) ;
#8582=CARTESIAN_POINT ( 'NONE',  ( -261.1919288306252724, -171.9377729149742038, -89.99999999999987210 ) ) ;
#8628=CARTESIAN_POINT ( 'NONE',  ( -261.1919288306253293, -171.9377729149742038, -104.9999999999998721 ) ) ;
#8642=EDGE_LOOP ( 'NONE', ( #24380, #20477, #27828, #15741 ) ) ;
#8656=DIRECTION ( 'NONE',  ( 2.775557561562887407E-16, 3.668437989309015303E-32, 1.000000000000000000 ) ) ;
#8659=CARTESIAN_POINT ( 'NONE',  ( -211.9745545450854536, -220.0000000000000853, -106.5998536507705552 ) ) ;
#8665=ADVANCED_FACE ( 'NONE', ( #25790 ), #1659, .T. ) ;
#8675=EDGE_CURVE ( 'NONE', #12396, #6070, #12459, .T. ) ;
#8688=AXIS2_PLACEMENT_3D ( 'NONE', #18845, #23018, #12542 ) ;
#8714=CARTESIAN_POINT ( 'NONE',  ( -213.1553235149935119, -216.8625818770119338, 94.90660418304274515 ) ) ;
#8730=DIRECTION ( 'NONE',  ( 0.8706753206611566043, 0.000000000000000000, -0.4918581970360891842 ) ) ;
#8748=VECTOR ( 'NONE', #1508, 1000.000000000000000 ) ;
#8757=CYLINDRICAL_SURFACE ( 'NONE', #3103, 67.21503689626328537 ) ;
#8779=VERTEX_POINT ( 'NONE', #4654 ) ;
#8793=CARTESIAN_POINT ( 'NONE',  ( -211.5426265866423989, -220.0000000000000853, -107.5190003421799645 ) ) ;
#8803=ORIENTED_EDGE ( 'NONE', *, *, #6323, .F. ) ;
#8835=CARTESIAN_POINT ( 'NONE',  ( -260.0000000000001137, -165.0000000000001137, -59.99999999999986500 ) ) ;
#8840=ORIENTED_EDGE ( 'NONE', *, *, #2019, .T. ) ;
#8843=CIRCLE ( 'NONE', #26722, 5.000000000000004441 ) ;
#8859=CYLINDRICAL_SURFACE ( 'NONE', #14927, 5.000000000000004441 ) ;
#8888=CARTESIAN_POINT ( 'NONE',  ( -279.1278187736259611, -165.0000000000001421, 106.1966075482099399 ) ) ;
#8893=DIRECTION ( 'NONE',  ( 1.000000000000000000, 0.000000000000000000, 0.000000000000000000 ) ) ;
#8904=DIRECTION ( 'NONE',  ( 1.000000000000000000, 0.000000000000000000, 0.000000000000000000 ) ) ;
#8933=DIRECTION ( 'NONE',  ( 0.000000000000000000, 0.000000000000000000, -1.000000000000000000 ) ) ;
#8939=DIRECTION ( 'NONE',  ( -1.000000000000000000, 5.551115123125784674E-16, 0.000000000000000000 ) ) ;
#8959=CIRCLE ( 'NONE', #8513, 34.99999999999997868 ) ;
#8963=AXIS2_PLACEMENT_3D ( 'NONE', #4264, #2104, #10883 ) ;
#9003=CARTESIAN_POINT ( 'NONE',  ( -277.2150368962633706, -170.0000000000001137, 90.47363622314041720 ) ) ;
#9109=ORIENTED_EDGE ( 'NONE', *, *, #22755, .F. ) ;
#9151=FACE_OUTER_BOUND ( 'NONE', #16856, .T. ) ;
#9169=ORIENTED_EDGE ( 'NONE', *, *, #27631, .F. ) ;
#9183=VECTOR ( 'NONE', #24514, 1000.000000000000000 ) ;
#9226=CARTESIAN_POINT ( 'NONE',  ( -290.0000000000001705, -165.0000000000001137, -59.99999999999986500 ) ) ;
#9229=LINE ( 'NONE', #17990, #7968 ) ;
#9246=CARTESIAN_POINT ( 'NONE',  ( -260.0000000000001137, -157.0000000000000284, 110.0000000000000142 ) ) ;
#9252=CARTESIAN_POINT ( 'NONE',  ( -268.8295757390185940, -165.3167864666411901, -88.70020982224049533 ) ) ;
#9256=EDGE_CURVE ( 'NONE', #301, #22565, #18924, .T. ) ;
#9305=B_SPLINE_CURVE_WITH_KNOTS ( 'NONE', 3,
 ( #1495, #14869, #5669, #23334, #25617, #5526 ),
 .UNSPECIFIED., .F., .F.,
 ( 4, 2, 4 ),
 ( 0.000000000000000000, 0.004615224477119865554, 0.009230448954239731107 ),
 .UNSPECIFIED. ) ;
#9314=AXIS2_PLACEMENT_3D ( 'NONE', #3248, #16349, #3529 ) ;
#9348=EDGE_LOOP ( 'NONE', ( #18552, #18045, #17219, #24251 ) ) ;
#9352=DIRECTION ( 'NONE',  ( -1.000000000000000000, 0.000000000000000000, 2.775557561562887407E-16 ) ) ;
#9403=CARTESIAN_POINT ( 'NONE',  ( -266.9577532651693446, -165.5716054493118463, -89.18913380684575998 ) ) ;
#9421=TOROIDAL_SURFACE ( 'NONE', #3428, 35.00000000000000711, 5.000000000000000000 ) ;
#9462=VERTEX_POINT ( 'NONE', #690 ) ;
#9476=CARTESIAN_POINT ( 'NONE',  ( -261.1919288306253293, -171.9377729149742038, 105.0000000000000142 ) ) ;
#9488=VERTEX_POINT ( 'NONE', #7000 ) ;
#9496=EDGE_CURVE ( 'NONE', #5842, #10608, #6557, .T. ) ;
#9538=DIRECTION ( 'NONE',  ( -1.000000000000000000, 4.540956701092242152E-16, 0.000000000000000000 ) ) ;
#9563=CARTESIAN_POINT ( 'NONE',  ( -271.9747264835629608, -170.1913680348071409, -103.5087831302661812 ) ) ;
#9565=ADVANCED_FACE ( 'NONE', ( #5553 ), #22807, .T. ) ;
#9589=DIRECTION ( 'NONE',  ( 1.000000000000000000, 0.000000000000000000, -3.053113317719176147E-15 ) ) ;
#9628=EDGE_CURVE ( 'NONE', #3224, #24423, #7030, .T. ) ;
#9687=DIRECTION ( 'NONE',  ( 0.000000000000000000, 0.000000000000000000, -1.000000000000000000 ) ) ;
#9705=EDGE_LOOP ( 'NONE', ( #17071, #21972, #10371, #5507, #7445, #26213, #26647, #8840 ) ) ;
#9721=CARTESIAN_POINT ( 'NONE',  ( -263.9041850570887959, -171.3165909455712494, 104.9297054525729322 ) ) ;
#9736=CARTESIAN_POINT ( 'NONE',  ( -305.0000000000001137, -157.0000000000000284, 60.00000000000002842 ) ) ;
#9744=EDGE_CURVE ( 'NONE', #12291, #21738, #19411, .T. ) ;
#9746=CARTESIAN_POINT ( 'NONE',  ( -260.0000000000001137, -157.0000000000000284, 105.0000000000000142 ) ) ;
#9785=AXIS2_PLACEMENT_3D ( 'NONE', #20924, #2972, #20644 ) ;
#9805=ORIENTED_EDGE ( 'NONE', *, *, #3407, .F. ) ;
#9811=CARTESIAN_POINT ( 'NONE',  ( -260.0000000000001137, -220.0000000000000853, -59.99999999999986500 ) ) ;
#9819=DIRECTION ( 'NONE',  ( -2.775557561562887407E-16, -3.668437989309015303E-32, 1.000000000000000000 ) ) ;
#9833=DIRECTION ( 'NONE',  ( -0.000000000000000000, -1.000000000000000000, -0.000000000000000000 ) ) ;
#9846=EDGE_CURVE ( 'NONE', #10091, #20874, #26489, .T. ) ;
#9856=CARTESIAN_POINT ( 'NONE',  ( -261.1919288306253293, -171.9377729149742038, 95.00000000000004263 ) ) ;
#9885=ADVANCED_BREP_SHAPE_REPRESENTATION ( '', ( #27732, #10637 ), #6979 ) ;
#9894=AXIS2_PLACEMENT_3D ( 'NONE', #6516, #15012, #12860 ) ;
#9911=ORIENTED_EDGE ( 'NONE', *, *, #19623, .F. ) ;
#9932=CIRCLE ( 'NONE', #13145, 5.000000000000004441 ) ;
#9939=ORIENTED_EDGE ( 'NONE', *, *, #27561, .T. ) ;
#9947=CARTESIAN_POINT ( 'NONE',  ( -210.0000000000000853, -218.4793454996984394, -90.61920026979450427 ) ) ;
#9954=CARTESIAN_POINT ( 'NONE',  ( -260.0000000000001137, -152.0000000000000284, -94.99999999999987210 ) ) ;
#9970=FACE_OUTER_BOUND ( 'NONE', #16350, .T. ) ;
#9999=CARTESIAN_POINT ( 'NONE',  ( -277.2150368962633706, -170.0000000000001421, 101.5769467933889558 ) ) ;
#10008=FACE_OUTER_BOUND ( 'NONE', #11130, .T. ) ;
#10010=ORIENTED_EDGE ( 'NONE', *, *, #21676, .T. ) ;
#10014=EDGE_CURVE ( 'NONE', #25748, #12291, #12568, .T. ) ;
#10018=VERTEX_POINT ( 'NONE', #19155 ) ;
#10025=CARTESIAN_POINT ( 'NONE',  ( -210.0000000000000568, -220.0000000000000853, -90.87829376371895762 ) ) ;
#10064=DIRECTION ( 'NONE',  ( 0.000000000000000000, 0.000000000000000000, 1.000000000000000000 ) ) ;
#10091=VERTEX_POINT ( 'NONE', #3641 ) ;
#10103=EDGE_LOOP ( 'NONE', ( #23265, #17570, #25522, #10985, #9939 ) ) ;
#10105=DIRECTION ( 'NONE',  ( -0.000000000000000000, -0.000000000000000000, 1.000000000000000000 ) ) ;
#10155=DIRECTION ( 'NONE',  ( 0.000000000000000000, 1.000000000000000000, 0.000000000000000000 ) ) ;
#10173=CARTESIAN_POINT ( 'NONE',  ( -270.0681032424402588, -170.3775688406267363, 93.68413306229582815 ) ) ;
#10174=EDGE_CURVE ( 'NONE', #3224, #301, #17563, .T. ) ;
#10181=CARTESIAN_POINT ( 'NONE',  ( -210.0000000000000568, -152.0000000000000284, -110.0000000000000284 ) ) ;
#10218=ORIENTED_EDGE ( 'NONE', *, *, #21742, .T. ) ;
#10230=EDGE_CURVE ( 'NONE', #27270, #28324, #14316, .T. ) ;
#10234=DIRECTION ( 'NONE',  ( 0.3825563754725206378, 0.000000000000000000, -0.9239321509641971186 ) ) ;
#10240=DIRECTION ( 'NONE',  ( 4.625929269271489858E-16, 0.000000000000000000, 1.000000000000000000 ) ) ;
#10255=DIRECTION ( 'NONE',  ( -1.000000000000000000, 0.000000000000000000, 3.053113317719176147E-15 ) ) ;
#10259=ORIENTED_EDGE ( 'NONE', *, *, #24097, .F. ) ;
#10308=CARTESIAN_POINT ( 'NONE',  ( -266.3442505907551663, -165.6659793133063374, -89.32861420273920317 ) ) ;
#10371=ORIENTED_EDGE ( 'NONE', *, *, #6731, .T. ) ;
#10381=EDGE_LOOP ( 'NONE', ( #11892, #13889, #9169, #16869 ) ) ;
#10411=CARTESIAN_POINT ( 'NONE',  ( -290.0000000000001705, -220.0000000000000853, -59.99999999999986500 ) ) ;
#10426=DIRECTION ( 'NONE',  ( 1.000000000000000000, -0.000000000000000000, -0.000000000000000000 ) ) ;
#10432=CARTESIAN_POINT ( 'NONE',  ( -305.0000000000001137, -157.0000000000000284, -110.0000000000000284 ) ) ;
#10499=CARTESIAN_POINT ( 'NONE',  ( -276.2002749566882471, -169.9725357324242907, -107.3290005716923901 ) ) ;
#10512=CIRCLE ( 'NONE', #5937, 4.999999999999995559 ) ;
#10550=DIRECTION ( 'NONE',  ( 1.000000000000000000, 0.000000000000000000, 1.921731041659628380E-16 ) ) ;
#10569=CARTESIAN_POINT ( 'NONE',  ( -265.0337338324069947, -165.8360419968486781, 89.68688984748098392 ) ) ;
#10578=ORIENTED_EDGE ( 'NONE', *, *, #5032, .T. ) ;
#10585=ORIENTED_EDGE ( 'NONE', *, *, #5972, .F. ) ;
#10588=DIRECTION ( 'NONE',  ( 1.000000000000000000, 1.321694076934710155E-16, 0.000000000000000000 ) ) ;
#10591=CARTESIAN_POINT ( 'NONE',  ( -272.1219990905822215, -170.1806730287380844, -93.00535902404892852 ) ) ;
#10592=CARTESIAN_POINT ( 'NONE',  ( -268.6807300700924088, -170.5270201242149994, 88.72748730061762501 ) ) ;
#10596=CARTESIAN_POINT ( 'NONE',  ( -263.9672435214092729, -171.3034507378823719, -94.90501643659933961 ) ) ;
#10608=VERTEX_POINT ( 'NONE', #22841 ) ;
#10612=ADVANCED_FACE ( 'NONE', ( #18390 ), #20256, .T. ) ;
#10637=AXIS2_PLACEMENT_3D ( 'NONE', #25065, #2320, #14860 ) ;
#10655=ORIENTED_EDGE ( 'NONE', *, *, #16626, .T. ) ;
#10657=ORIENTED_EDGE ( 'NONE', *, *, #12227, .F. ) ;
#10665=CARTESIAN_POINT ( 'NONE',  ( -295.0000000000001137, -165.0000000000000853, 60.00000000000002842 ) ) ;
#10683=CARTESIAN_POINT ( 'NONE',  ( -210.0000000000000568, -220.0000000000000853, -110.0000000000000284 ) ) ;
#10701=AXIS2_PLACEMENT_3D ( 'NONE', #10722, #28221, #10155 ) ;
#10722=CARTESIAN_POINT ( 'NONE',  ( -210.0000000000000568, -157.0000000000000284, -105.0000000000000284 ) ) ;
#10725=B_SPLINE_CURVE_WITH_KNOTS ( 'NONE', 3,
 ( #12792, #21536, #12373, #1849, #7900, #21112, #3720, #1429 ),
 .UNSPECIFIED., .F., .F.,
 ( 4, 2, 2, 4 ),
 ( 0.000000000000000000, 0.009823278049383234872, 0.01473491707407493558, 0.01964655609876663628 ),
 .UNSPECIFIED. ) ;
#10727=CIRCLE ( 'NONE', #18070, 49.99999999999998579 ) ;
#10735=CARTESIAN_POINT ( 'NONE',  ( -212.3316009019935962, -218.3936534609811986, 93.13925850349481550 ) ) ;
#10740=CARTESIAN_POINT ( 'NONE',  ( -264.4418871519581558, -166.0055717401948527, -89.67623118319436060 ) ) ;
#10778=FACE_OUTER_BOUND ( 'NONE', #8642, .T. ) ;
#10789=ORIENTED_EDGE ( 'NONE', *, *, #2934, .T. ) ;
#10795=CIRCLE ( 'NONE', #25029, 29.99999999999998934 ) ;
#10804=CARTESIAN_POINT ( 'NONE',  ( -211.3305068427980871, -219.3267326664164614, 108.0785994798089433 ) ) ;
#10857=DIRECTION ( 'NONE',  ( -1.000000000000000000, 7.930164461608254523E-16, 0.000000000000000000 ) ) ;
#10860=AXIS2_PLACEMENT_3D ( 'NONE', #25073, #24932, #802 ) ;
#10862=ORIENTED_EDGE ( 'NONE', *, *, #25409, .T. ) ;
#10883=DIRECTION ( 'NONE',  ( 0.000000000000000000, 0.000000000000000000, -1.000000000000000000 ) ) ;
#10903=VERTEX_POINT ( 'NONE', #9856 ) ;
#10943=CARTESIAN_POINT ( 'NONE',  ( -213.0597602322720832, -217.1208202143830306, 105.3784789975249794 ) ) ;
#10951=DIRECTION ( 'NONE',  ( -2.775557561562887407E-16, -3.668437989309015850E-32, -1.000000000000000000 ) ) ;
#10960=SHAPE_REPRESENTATION_RELATIONSHIP ( 'NONE' , 'NONE' ,  #3128, #9885 ) ;
#10985=ORIENTED_EDGE ( 'NONE', *, *, #11177, .T. ) ;
#10997=CARTESIAN_POINT ( 'NONE',  ( -260.0000000000001137, -220.0000000000000853, -89.99999999999985789 ) ) ;
#11059=CARTESIAN_POINT ( 'NONE',  ( -260.0000000000001137, -152.0000000000000284, -59.99999999999986500 ) ) ;
#11087=AXIS2_PLACEMENT_3D ( 'NONE', #25478, #27760, #12000 ) ;
#11096=DIRECTION ( 'NONE',  ( 4.540956701092242152E-16, 1.000000000000000000, 0.000000000000000000 ) ) ;
#11116=PLANE ( 'NONE',  #9894 ) ;
#11130=EDGE_LOOP ( 'NONE', ( #27309, #25975, #21133, #27806 ) ) ;
#11148=EDGE_LOOP ( 'NONE', ( #14817, #7746, #8384, #11449, #14935, #22458, #5051, #23019, #24331, #16037, #2091, #618 ) ) ;
#11177=EDGE_CURVE ( 'NONE', #28358, #268, #16094, .T. ) ;
#11212=EDGE_CURVE ( 'NONE', #20874, #9488, #7490, .T. ) ;
#11231=CARTESIAN_POINT ( 'NONE',  ( -211.4917091876254744, -219.2061850725015120, 107.9125863485613195 ) ) ;
#11233=VECTOR ( 'NONE', #9589, 1000.000000000000000 ) ;
#11350=CARTESIAN_POINT ( 'NONE',  ( -260.0000000000001137, -157.0000000000000284, 60.00000000000002132 ) ) ;
#11397=DIRECTION ( 'NONE',  ( -1.321694076934710155E-16, 1.000000000000000000, 0.000000000000000000 ) ) ;
#11440=CARTESIAN_POINT ( 'NONE',  ( -270.6366141379085093, -170.3090574957601291, -103.8655989124723504 ) ) ;
#11449=ORIENTED_EDGE ( 'NONE', *, *, #19350, .T. ) ;
#11459=CARTESIAN_POINT ( 'NONE',  ( -275.9792957272333638, -170.0000000000001137, 91.22365543927794818 ) ) ;
#11468=DIRECTION ( 'NONE',  ( -1.000000000000000000, 0.000000000000000000, 0.000000000000000000 ) ) ;
#11488=CARTESIAN_POINT ( 'NONE',  ( -260.0000000000001137, -152.0000000000000284, 95.00000000000000000 ) ) ;
#11489=EDGE_CURVE ( 'NONE', #6860, #27270, #19875, .T. ) ;
#11538=CARTESIAN_POINT ( 'NONE',  ( -210.0000000000000568, -152.0000000000000284, 105.0000000000000284 ) ) ;
#11542=AXIS2_PLACEMENT_3D ( 'NONE', #21838, #23705, #2143 ) ;
#11572=LINE ( 'NONE', #211, #26312 ) ;
#11580=EDGE_LOOP ( 'NONE', ( #25097, #18556, #3845, #27592, #20783 ) ) ;
#11598=ORIENTED_EDGE ( 'NONE', *, *, #16469, .T. ) ;
#11646=FACE_OUTER_BOUND ( 'NONE', #21999, .T. ) ;
#11661=AXIS2_PLACEMENT_3D ( 'NONE', #7731, #20657, #22958 ) ;
#11682=AXIS2_PLACEMENT_3D ( 'NONE', #18685, #16266, #16126 ) ;
#11699=CARTESIAN_POINT ( 'NONE',  ( -260.0000000000001137, -157.0000000000000284, -59.99999999999986500 ) ) ;
#11715=CARTESIAN_POINT ( 'NONE',  ( -277.2150368962633706, -237.2150368962634559, 95.00000000000004263 ) ) ;
#11718=CIRCLE ( 'NONE', #24533, 5.000000000000004441 ) ;
#11742=ADVANCED_FACE ( 'NONE', ( #7427 ), #23214, .T. ) ;
#11753=CARTESIAN_POINT ( 'NONE',  ( -261.1919288306253293, -171.9377729149742038, 110.0000000000000142 ) ) ;
#11793=ORIENTED_EDGE ( 'NONE', *, *, #24931, .F. ) ;
#11813=AXIS2_PLACEMENT_3D ( 'NONE', #8006, #20934, #14339 ) ;
#11845=CARTESIAN_POINT ( 'NONE',  ( -273.6138116763045787, -165.0000000000001990, -86.76535624830611937 ) ) ;
#11852=DIRECTION ( 'NONE',  ( -0.000000000000000000, -1.000000000000000000, -0.000000000000000000 ) ) ;
#11858=DIRECTION ( 'NONE',  ( 0.000000000000000000, 0.000000000000000000, -1.000000000000000000 ) ) ;
#11865=AXIS2_PLACEMENT_3D ( 'NONE', #9736, #22944, #22378 ) ;
#11873=VECTOR ( 'NONE', #3520, 1000.000000000000000 ) ;
#11892=ORIENTED_EDGE ( 'NONE', *, *, #13513, .T. ) ;
#11913=CARTESIAN_POINT ( 'NONE',  ( -211.4334854057310338, -220.0000000000001421, -92.30784275734241362 ) ) ;
#11917=FACE_OUTER_BOUND ( 'NONE', #17407, .T. ) ;
#12000=DIRECTION ( 'NONE',  ( -1.000000000000000000, 0.000000000000000000, 3.097027491608645765E-15 ) ) ;
#12010=EDGE_CURVE ( 'NONE', #3702, #22223, #11572, .T. ) ;
#12024=CARTESIAN_POINT ( 'NONE',  ( -266.6333112347296606, -170.8236892866178209, 104.6429431552469111 ) ) ;
#12027=DIRECTION ( 'NONE',  ( -1.000000000000000000, -1.321694076934710155E-16, 0.000000000000000000 ) ) ;
#12035=DIRECTION ( 'NONE',  ( -1.000000000000000000, 0.000000000000000000, -2.775557561562887407E-16 ) ) ;
#12086=AXIS2_PLACEMENT_3D ( 'NONE', #15347, #25818, #24103 ) ;
#12120=AXIS2_PLACEMENT_3D ( 'NONE', #19946, #2556, #8893 ) ;
#12134=( BOUNDED_SURFACE ( )  B_SPLINE_SURFACE ( 3, 2, ( 
 ( #3545, #6136, #27951 ),
 ( #12337, #27671, #5849 ),
 ( #21647, #14912, #14620 ),
 ( #10591, #23666, #23378 ),
 ( #25667, #14767, #3972 ),
 ( #21498, #12478, #3686 ),
 ( #21219, #1817, #10308 ),
 ( #5712, #21079, #19067 ),
 ( #1957, #19347, #10740 ),
 ( #25954, #28096, #8440 ),
 ( #4115, #5990, #28237 ),
 ( #19494, #8582, #23519 ) ),
 .UNSPECIFIED., .F., .F., .T. ) 
 B_SPLINE_SURFACE_WITH_KNOTS ( ( 4, 2, 2, 2, 2, 4 ),
 ( 3, 3 ),
 ( 0.000000000000000000, 0.004509347248874698982, 0.009018694497749397965, 0.01127336812218674746, 0.01352804174662409695, 0.01803738899549879593 ),
 ( 0.000000000000000000, 1.000000000000000000 ),
 .UNSPECIFIED. ) 
 GEOMETRIC_REPRESENTATION_ITEM ( )  RATIONAL_B_SPLINE_SURFACE ( (
 ( 1.000000000000000000, 0.7071067811865466846, 1.000000000000000000),
 ( 1.000000000000000000, 0.7039097745451907695, 1.000000000000000000),
 ( 1.000000000000000000, 0.7013522928558304503, 1.000000000000000000),
 ( 1.000000000000000000, 0.6977882347214663383, 1.000000000000000000),
 ( 1.000000000000000000, 0.6967820801478910031, 1.000000000000000000),
 ( 1.000000000000000000, 0.6966221438781953212, 1.000000000000000000),
 ( 1.000000000000000000, 0.6967948695995229702, 1.000000000000000000),
 ( 1.000000000000000000, 0.6976115817203014657, 1.000000000000000000),
 ( 1.000000000000000000, 0.6982527460775038719, 1.000000000000000000),
 ( 1.000000000000000000, 0.7008698237985928614, 1.000000000000000000),
 ( 1.000000000000000000, 0.7035399889988015465, 1.000000000000000000),
 ( 1.000000000000000000, 0.7071067811865475727, 1.000000000000000000) ) ) 
 REPRESENTATION_ITEM ( '' )  SURFACE ( )  );
#12137=CARTESIAN_POINT ( 'NONE',  ( -260.0000000000001137, -157.0000000000000284, 60.00000000000002132 ) ) ;
#12158=ORIENTED_EDGE ( 'NONE', *, *, #1590, .F. ) ;
#12169=CARTESIAN_POINT ( 'NONE',  ( -266.4957295474704893, -165.8849619812661444, 109.6032701725642937 ) ) ;
#12186=VECTOR ( 'NONE', #4823, 1000.000000000000000 ) ;
#12227=EDGE_CURVE ( 'NONE', #22223, #23150, #10727, .T. ) ;
#12242=AXIS2_PLACEMENT_3D ( 'NONE', #27724, #8065, #7921 ) ;
#12248=ORIENTED_EDGE ( 'NONE', *, *, #20192, .T. ) ;
#12268=FACE_OUTER_BOUND ( 'NONE', #14603, .T. ) ;
#12280=DIRECTION ( 'NONE',  ( -3.053113317719176147E-15, -4.035281788239917819E-31, -1.000000000000000000 ) ) ;
#12291=VERTEX_POINT ( 'NONE', #18861 ) ;
#12311=DIRECTION ( 'NONE',  ( 1.321694076934710155E-16, -1.000000000000000000, 0.000000000000000000 ) ) ;
#12317=CARTESIAN_POINT ( 'NONE',  ( -277.2150368962633706, -170.0000000000001137, -110.0000000000000284 ) ) ;
#12337=CARTESIAN_POINT ( 'NONE',  ( -275.9795250186070916, -170.0000000000001137, -91.22351627327833512 ) ) ;
#12340=CARTESIAN_POINT ( 'NONE',  ( -266.9750954100557010, -170.7663605388744941, 89.20968119495026372 ) ) ;
#12373=CARTESIAN_POINT ( 'NONE',  ( -266.4635733393146779, -165.8461665555755076, -109.6876586681348584 ) ) ;
#12377=CIRCLE ( 'NONE', #28393, 5.000000000000000888 ) ;
#12386=CARTESIAN_POINT ( 'NONE',  ( -277.6780266850147427, -169.9634972840153466, -106.7968975218380763 ) ) ;
#12396=VERTEX_POINT ( 'NONE', #23884 ) ;
#12417=EDGE_LOOP ( 'NONE', ( #15251, #20649, #15366, #23754 ) ) ;
#12430=CARTESIAN_POINT ( 'NONE',  ( -210.0000000000000568, -220.0000000000000853, -110.0000000000000284 ) ) ;
#12459=LINE ( 'NONE', #12317, #21646 ) ;
#12466=EDGE_LOOP ( 'NONE', ( #5022, #19923, #10259, #19513 ) ) ;
#12472=CARTESIAN_POINT ( 'NONE',  ( -260.0000000000001137, -220.0000000000000853, 60.00000000000002132 ) ) ;
#12478=CARTESIAN_POINT ( 'NONE',  ( -267.5881315349600982, -170.6799793700724877, -89.03726891381465691 ) ) ;
#12527=AXIS2_PLACEMENT_3D ( 'NONE', #12472, #3969, #10588 ) ;
#12542=DIRECTION ( 'NONE',  ( 1.000000000000000000, 0.000000000000000000, -2.064684994405763843E-16 ) ) ;
#12565=EDGE_LOOP ( 'NONE', ( #18875, #3078, #3780, #26515 ) ) ;
#12568=LINE ( 'NONE', #10683, #15690 ) ;
#12599=FACE_OUTER_BOUND ( 'NONE', #12466, .T. ) ;
#12600=DIRECTION ( 'NONE',  ( -1.000000000000000000, -0.000000000000000000, 3.053113317719176147E-15 ) ) ;
#12619=ADVANCED_FACE ( 'NONE', ( #3306 ), #14415, .T. ) ;
#12640=VERTEX_POINT ( 'NONE', #20418 ) ;
#12657=CARTESIAN_POINT ( 'NONE',  ( -210.0000000000000568, -157.0000000000000284, 105.0000000000000284 ) ) ;
#12662=CARTESIAN_POINT ( 'NONE',  ( -210.0000000000000568, -152.0000000000000284, -94.99999999999987210 ) ) ;
#12663=DIRECTION ( 'NONE',  ( -1.321694076934710155E-16, 1.000000000000000000, 0.000000000000000000 ) ) ;
#12683=DIRECTION ( 'NONE',  ( -4.625929269271489858E-16, 0.000000000000000000, -1.000000000000000000 ) ) ;
#12688=EDGE_CURVE ( 'NONE', #5617, #25077, #27163, .T. ) ;
#12741=DIRECTION ( 'NONE',  ( -0.000000000000000000, -0.000000000000000000, 1.000000000000000000 ) ) ;
#12760=CARTESIAN_POINT ( 'NONE',  ( -263.5350310235390339, -171.3954706173032321, 89.83034331963602881 ) ) ;
#12781=VECTOR ( 'NONE', #2687, 1000.000000000000000 ) ;
#12792=CARTESIAN_POINT ( 'NONE',  ( -260.0000000000001137, -167.0819201924624906, -109.9999999999998721 ) ) ;
#12820=DIRECTION ( 'NONE',  ( 1.000000000000000000, 1.321694076934710155E-16, -4.625929269271489858E-16 ) ) ;
#12860=DIRECTION ( 'NONE',  ( -1.321694076934710155E-16, 1.000000000000000000, 0.000000000000000000 ) ) ;
#12886=CARTESIAN_POINT ( 'NONE',  ( -270.1042321369618548, -170.3737068505718639, 93.67314610463054692 ) ) ;
#12901=CARTESIAN_POINT ( 'NONE',  ( -268.7977277042236892, -165.3316741299294392, 88.68837795047839734 ) ) ;
#12938=DIRECTION ( 'NONE',  ( 0.000000000000000000, 1.000000000000000000, 0.000000000000000000 ) ) ;
#12947=CARTESIAN_POINT ( 'NONE',  ( -272.8482960613322348, -165.2072238553256227, -108.3495407332041651 ) ) ;
#12953=EDGE_CURVE ( 'NONE', #301, #12291, #2532, .T. ) ;
#12958=CIRCLE ( 'NONE', #5157, 72.21503689626329958 ) ;
#12984=AXIS2_PLACEMENT_3D ( 'NONE', #18101, #13804, #7326 ) ;
#12995=ORIENTED_EDGE ( 'NONE', *, *, #6567, .F. ) ;
#13028=CIRCLE ( 'NONE', #630, 4.999999999999992895 ) ;
#13042=CARTESIAN_POINT ( 'NONE',  ( -211.7958164186347574, -218.9496041985363490, 92.43018420650685130 ) ) ;
#13115=CARTESIAN_POINT ( 'NONE',  ( -210.4359063544881394, -219.8547609215023897, 108.8564660827533999 ) ) ;
#13145=AXIS2_PLACEMENT_3D ( 'NONE', #4739, #20113, #13668 ) ;
#13160=CARTESIAN_POINT ( 'NONE',  ( -290.0000000000001137, -157.0000000000000284, 60.00000000000002842 ) ) ;
#13170=EDGE_LOOP ( 'NONE', ( #8051, #13510, #8803, #12995 ) ) ;
#13171=ADVANCED_FACE ( 'NONE', ( #12599 ), #1583, .T. ) ;
#13212=FACE_OUTER_BOUND ( 'NONE', #27661, .T. ) ;
#13251=EDGE_CURVE ( 'NONE', #17075, #3368, #8031, .T. ) ;
#13287=CARTESIAN_POINT ( 'NONE',  ( -260.0000000000001137, -157.0000000000000284, -94.99999999999985789 ) ) ;
#13297=AXIS2_PLACEMENT_3D ( 'NONE', #17660, #17799, #26555 ) ;
#13323=DIRECTION ( 'NONE',  ( -0.000000000000000000, -0.000000000000000000, 1.000000000000000000 ) ) ;
#13337=ORIENTED_EDGE ( 'NONE', *, *, #3451, .T. ) ;
#13368=EDGE_LOOP ( 'NONE', ( #24336, #5132, #13703, #15566 ) ) ;
#13386=CARTESIAN_POINT ( 'NONE',  ( -212.5524510162168212, -218.0941723687617184, 106.4974602408248074 ) ) ;
#13393=ADVANCED_FACE ( 'NONE', ( #9970 ), #9421, .T. ) ;
#13397=DIRECTION ( 'NONE',  ( 1.000000000000000000, 0.000000000000000000, -1.921731041659628380E-16 ) ) ;
#13400=CARTESIAN_POINT ( 'NONE',  ( -210.0000000000000568, -220.0000000000000853, -109.1217062362807155 ) ) ;
#13412=ORIENTED_EDGE ( 'NONE', *, *, #5748, .F. ) ;
#13434=DIRECTION ( 'NONE',  ( 4.625929269271489858E-16, -0.000000000000000000, 1.000000000000000000 ) ) ;
#13445=CARTESIAN_POINT ( 'NONE',  ( -272.7817474293340183, -170.1432013118196380, 92.71875118442027031 ) ) ;
#13461=CARTESIAN_POINT ( 'NONE',  ( -213.1827219047386848, -216.7767438708612531, 105.0000000000000142 ) ) ;
#13463=CARTESIAN_POINT ( 'NONE',  ( -272.4467628956543876, -165.0365710123801648, 87.32694055142955847 ) ) ;
#13471=VECTOR ( 'NONE', #8075, 1000.000000000000000 ) ;
#13510=ORIENTED_EDGE ( 'NONE', *, *, #24935, .F. ) ;
#13513=EDGE_CURVE ( 'NONE', #5554, #28289, #1603, .T. ) ;
#13525=VERTEX_POINT ( 'NONE', #27894 ) ;
#13530=VERTEX_POINT ( 'NONE', #6077 ) ;
#13533=CARTESIAN_POINT ( 'NONE',  ( -212.8298628423295895, -217.6190342207067374, 105.9424056457623777 ) ) ;
#13611=LINE ( 'NONE', #24365, #12186 ) ;
#13650=FACE_OUTER_BOUND ( 'NONE', #13368, .T. ) ;
#13668=DIRECTION ( 'NONE',  ( -1.000000000000000000, 0.000000000000000000, 0.000000000000000000 ) ) ;
#13692=ORIENTED_EDGE ( 'NONE', *, *, #24931, .T. ) ;
#13698=ORIENTED_EDGE ( 'NONE', *, *, #18052, .T. ) ;
#13703=ORIENTED_EDGE ( 'NONE', *, *, #20192, .F. ) ;
#13723=CARTESIAN_POINT ( 'NONE',  ( -295.0000000000002274, -152.0000000000000284, -59.99999999999986500 ) ) ;
#13749=EDGE_CURVE ( 'NONE', #17968, #10903, #17683, .T. ) ;
#13750=AXIS2_PLACEMENT_3D ( 'NONE', #8232, #3491, #21437 ) ;
#13775=CARTESIAN_POINT ( 'NONE',  ( -310.0000000000001137, -157.0000000000000284, -59.99999999999987210 ) ) ;
#13789=UNCERTAINTY_MEASURE_WITH_UNIT (LENGTH_MEASURE( 1.000000000000000082E-05 ), #15284, 'distance_accuracy_value', 'NONE');
#13804=DIRECTION ( 'NONE',  ( 1.000000000000000000, 0.000000000000000000, 0.000000000000000000 ) ) ;
#13816=ORIENTED_EDGE ( 'NONE', *, *, #14231, .F. ) ;
#13860=CARTESIAN_POINT ( 'NONE',  ( -338.3377857851766635, -170.0000000000000853, -110.0000000000000284 ) ) ;
#13864=CARTESIAN_POINT ( 'NONE',  ( -261.2610864772255468, -166.7207794580371853, -89.99999999999990052 ) ) ;
#13889=ORIENTED_EDGE ( 'NONE', *, *, #20063, .F. ) ;
#13908=CARTESIAN_POINT ( 'NONE',  ( -262.6917462842096143, -171.5696242569879075, 109.9616379985420167 ) ) ;
#13948=ADVANCED_FACE ( 'NONE', ( #27718 ), #7347, .T. ) ;
#13997=EDGE_LOOP ( 'NONE', ( #27276, #22644, #25298, #23301, #26606, #1701, #18946, #13337 ) ) ;
#13998=FACE_OUTER_BOUND ( 'NONE', #27373, .T. ) ;
#14047=CARTESIAN_POINT ( 'NONE',  ( -268.1131488955604141, -165.6689427093874372, 109.3643454197753897 ) ) ;
#14205=CIRCLE ( 'NONE', #8218, 4.999999999999995559 ) ;
#14211=CARTESIAN_POINT ( 'NONE',  ( -210.0000000000000568, -210.8114316696540982, 90.00000000000002842 ) ) ;
#14231=EDGE_CURVE ( 'NONE', #5806, #3147, #18996, .T. ) ;
#14270=CARTESIAN_POINT ( 'NONE',  ( -210.0000000000000568, -220.0000000000000853, -109.1217062362807155 ) ) ;
#14272=VECTOR ( 'NONE', #5295, 1000.000000000000000 ) ;
#14290=ADVANCED_FACE ( 'NONE', ( #18712 ), #1468, .T. ) ;
#14304=ORIENTED_EDGE ( 'NONE', *, *, #9256, .F. ) ;
#14305=EDGE_LOOP ( 'NONE', ( #4138, #24523, #21272, #2686, #5305 ) ) ;
#14315=CARTESIAN_POINT ( 'NONE',  ( -272.0101343024082325, -170.1474602875829589, 103.5721376568295256 ) ) ;
#14316=CIRCLE ( 'NONE', #20718, 5.000000000000004441 ) ;
#14334=AXIS2_PLACEMENT_3D ( 'NONE', #4608, #8656, #4757 ) ;
#14339=DIRECTION ( 'NONE',  ( -1.000000000000000000, 0.000000000000000000, 0.000000000000000000 ) ) ;
#14349=CARTESIAN_POINT ( 'NONE',  ( -270.8397870484705550, -170.2891267554672936, -93.46372687881502372 ) ) ;
#14379=DIRECTION ( 'NONE',  ( -1.000000000000000000, 0.000000000000000000, 0.000000000000000000 ) ) ;
#14381=CARTESIAN_POINT ( 'NONE',  ( -210.0000000000000568, -157.0000000000000284, -89.99999999999987210 ) ) ;
#14415=TOROIDAL_SURFACE ( 'NONE', #11682, 72.21503689626331379, 5.000000000000000000 ) ;
#14488=CARTESIAN_POINT ( 'NONE',  ( -270.0328369100889745, -165.2068861618994902, 88.28012068083718589 ) ) ;
#14544=ORIENTED_EDGE ( 'NONE', *, *, #11212, .F. ) ;
#14556=PLANE ( 'NONE',  #15972 ) ;
#14587=DIRECTION ( 'NONE',  ( -1.321694076934710155E-16, 1.000000000000000000, 0.000000000000000000 ) ) ;
#14603=EDGE_LOOP ( 'NONE', ( #2785, #24898, #9805, #4582 ) ) ;
#14620=CARTESIAN_POINT ( 'NONE',  ( -272.4516753896481873, -165.0365817940426325, -87.32421121213782556 ) ) ;
#14654=CIRCLE ( 'NONE', #4528, 49.99999999999998579 ) ;
#14655=AXIS2_PLACEMENT_3D ( 'NONE', #11699, #2621, #16143 ) ;
#14667=CARTESIAN_POINT ( 'NONE',  ( -279.1278187736259611, -170.0000000000001137, -106.1966075482098262 ) ) ;
#14691=DIRECTION ( 'NONE',  ( -1.321694076934710155E-16, 1.000000000000000000, 0.000000000000000000 ) ) ;
#14746=CARTESIAN_POINT ( 'NONE',  ( -260.0000000000001137, -152.0000000000000284, -104.9999999999998721 ) ) ;
#14767=CARTESIAN_POINT ( 'NONE',  ( -269.2930304670530290, -170.4418591343095386, -88.55248351026435216 ) ) ;
#14768=CARTESIAN_POINT ( 'NONE',  ( -260.0000000000001137, -167.0819201924624906, 110.0000000000000142 ) ) ;
#14773=DIRECTION ( 'NONE',  ( 3.053113317719176147E-15, 4.035281788239917819E-31, 1.000000000000000000 ) ) ;
#14817=ORIENTED_EDGE ( 'NONE', *, *, #2472, .F. ) ;
#14827=ORIENTED_EDGE ( 'NONE', *, *, #16661, .T. ) ;
#14854=ORIENTED_EDGE ( 'NONE', *, *, #12953, .T. ) ;
#14859=ORIENTED_EDGE ( 'NONE', *, *, #16178, .T. ) ;
#14860=DIRECTION ( 'NONE',  ( 1.000000000000000000, 0.000000000000000000, 0.000000000000000000 ) ) ;
#14869=CARTESIAN_POINT ( 'NONE',  ( -210.0000000000000000, -218.4793454996983826, -109.3807997302051973 ) ) ;
#14912=CARTESIAN_POINT ( 'NONE',  ( -272.6023736344520785, -170.1165736173990695, -87.25084524916873363 ) ) ;
#14913=CARTESIAN_POINT ( 'NONE',  ( -261.1919288306252724, -171.9377729149742038, 90.00000000000001421 ) ) ;
#14927=AXIS2_PLACEMENT_3D ( 'NONE', #20201, #20053, #17905 ) ;
#14931=EDGE_LOOP ( 'NONE', ( #19059, #2542, #790, #27378, #10862 ) ) ;
#14935=ORIENTED_EDGE ( 'NONE', *, *, #24536, .T. ) ;
#15012=DIRECTION ( 'NONE',  ( 1.000000000000000000, 1.321694076934710155E-16, 0.000000000000000000 ) ) ;
#15028=CARTESIAN_POINT ( 'NONE',  ( -270.6285134702751520, -165.1572588087801421, 88.06168287673186512 ) ) ;
#15038=DIRECTION ( 'NONE',  ( -1.321694076934710155E-16, 1.000000000000000000, 0.000000000000000000 ) ) ;
#15050=CARTESIAN_POINT ( 'NONE',  ( -265.8373424361719799, -170.9544065693361290, 89.46035631147101697 ) ) ;
#15100=CARTESIAN_POINT ( 'NONE',  ( -277.5909579262273041, -164.9999999998546798, -106.8329485552555269 ) ) ;
#15114=DIRECTION ( 'NONE',  ( 1.000000000000000000, 0.000000000000000000, 0.000000000000000000 ) ) ;
#15180=CARTESIAN_POINT ( 'NONE',  ( -266.5073747506846189, -165.8832655043242994, 109.6017926887263343 ) ) ;
#15191=CARTESIAN_POINT ( 'NONE',  ( -212.8298628423295895, -217.6190342207067943, 94.05759435423763648 ) ) ;
#15195=CARTESIAN_POINT ( 'NONE',  ( -273.6825128178298883, -170.0454220111860764, 86.72654589157289706 ) ) ;
#15232=CARTESIAN_POINT ( 'NONE',  ( -210.0000000000000568, -210.8114316696540982, -89.99999999999987210 ) ) ;
#15251=ORIENTED_EDGE ( 'NONE', *, *, #22635, .T. ) ;
#15284=( LENGTH_UNIT ( ) NAMED_UNIT ( * ) SI_UNIT ( .MILLI., .METRE. ) );
#15288=DIRECTION ( 'NONE',  ( 1.000000000000000000, 0.000000000000000000, 0.000000000000000000 ) ) ;
#15317=CARTESIAN_POINT ( 'NONE',  ( -268.7788207492064316, -165.3337907801079325, 88.69420594919965595 ) ) ;
#15318=DIRECTION ( 'NONE',  ( 1.000000000000000000, 0.000000000000000000, 2.064684994405763843E-16 ) ) ;
#15321=VERTEX_POINT ( 'NONE', #27329 ) ;
#15332=ORIENTED_EDGE ( 'NONE', *, *, #18595, .T. ) ;
#15344=CARTESIAN_POINT ( 'NONE',  ( -274.7382056584871748, -170.0332543031711339, -91.86557292422580190 ) ) ;
#15347=CARTESIAN_POINT ( 'NONE',  ( -260.0000000000001137, -157.0000000000000284, -59.99999999999986500 ) ) ;
#15356=APPLICATION_CONTEXT ( 'automotive_design' ) ;
#15366=ORIENTED_EDGE ( 'NONE', *, *, #21846, .F. ) ;
#15419=CARTESIAN_POINT ( 'NONE',  ( -210.3420462306316949, -220.0000000000000853, -108.8941602138125262 ) ) ;
#15464=EDGE_CURVE ( 'NONE', #28358, #5554, #23596, .T. ) ;
#15482=CARTESIAN_POINT ( 'NONE',  ( -273.6177394993287635, -164.9999999998519797, 86.76313735923795889 ) ) ;
#15491=CARTESIAN_POINT ( 'NONE',  ( -277.2150368962633706, -165.0000000000001137, -90.47363622314027509 ) ) ;
#15521=EDGE_CURVE ( 'NONE', #5806, #21087, #21459, .T. ) ;
#15542=ORIENTED_EDGE ( 'NONE', *, *, #9744, .T. ) ;
#15552=FACE_OUTER_BOUND ( 'NONE', #7402, .T. ) ;
#15556=CARTESIAN_POINT ( 'NONE',  ( -212.2419371577844913, -220.0000000000001137, -105.4110757242456771 ) ) ;
#15566=ORIENTED_EDGE ( 'NONE', *, *, #24570, .F. ) ;
#15579=CARTESIAN_POINT ( 'NONE',  ( -266.6560114757872952, -170.8199632925098115, 104.6399347438232894 ) ) ;
#15606=CARTESIAN_POINT ( 'NONE',  ( -277.2150368962633706, -170.0000000000001137, 90.47363622314043141 ) ) ;
#15654=VECTOR ( 'NONE', #12663, 1000.000000000000000 ) ;
#15690=VECTOR ( 'NONE', #1762, 1000.000000000000000 ) ;
#15697=CARTESIAN_POINT ( 'NONE',  ( -277.2150368962633706, -237.2150368962634559, -89.99999999999985789 ) ) ;
#15736=DIRECTION ( 'NONE',  ( -1.000000000000000000, 0.000000000000000000, 0.000000000000000000 ) ) ;
#15741=ORIENTED_EDGE ( 'NONE', *, *, #5146, .F. ) ;
#15746=DIRECTION ( 'NONE',  ( -0.000000000000000000, -1.000000000000000000, -0.000000000000000000 ) ) ;
#15774=CARTESIAN_POINT ( 'NONE',  ( -290.0000000000001705, -165.0000000000001137, -59.99999999999986500 ) ) ;
#15831=ORIENTED_EDGE ( 'NONE', *, *, #11177, .F. ) ;
#15855=ORIENTED_EDGE ( 'NONE', *, *, #27561, .F. ) ;
#15867=ORIENTED_EDGE ( 'NONE', *, *, #18052, .F. ) ;
#15897=CARTESIAN_POINT ( 'NONE',  ( -277.2150368962633706, -170.0000000000001137, -101.5769467933888137 ) ) ;
#15912=DIRECTION ( 'NONE',  ( 0.000000000000000000, 0.000000000000000000, -1.000000000000000000 ) ) ;
#15942=CARTESIAN_POINT ( 'NONE',  ( -295.0000000000001137, -157.0000000000000284, 60.00000000000002842 ) ) ;
#15944=ADVANCED_FACE ( 'NONE', ( #6736 ), #17093, .T. ) ;
#15971=LINE ( 'NONE', #27149, #3073 ) ;
#15972=AXIS2_PLACEMENT_3D ( 'NONE', #28021, #16709, #1469 ) ;
#15987=DIRECTION ( 'NONE',  ( -0.000000000000000000, -0.000000000000000000, 1.000000000000000000 ) ) ;
#15990=AXIS2_PLACEMENT_3D ( 'NONE', #11350, #22400, #22253 ) ;
#16014=CARTESIAN_POINT ( 'NONE',  ( -266.3253780546114626, -165.6690032019043599, -89.33268690869475392 ) ) ;
#16029=EDGE_LOOP ( 'NONE', ( #25906, #9911, #7146, #6722, #26713 ) ) ;
#16037=ORIENTED_EDGE ( 'NONE', *, *, #24060, .T. ) ;
#16070=ORIENTED_EDGE ( 'NONE', *, *, #26101, .F. ) ;
#16094=LINE ( 'NONE', #2419, #16212 ) ;
#16113=AXIS2_PLACEMENT_3D ( 'NONE', #2676, #21937, #11468 ) ;
#16126=DIRECTION ( 'NONE',  ( 1.000000000000000000, 3.004539147878382249E-48, 2.775557561562887407E-16 ) ) ;
#16127=ORIENTED_EDGE ( 'NONE', *, *, #24935, .T. ) ;
#16143=DIRECTION ( 'NONE',  ( 0.000000000000000000, 0.000000000000000000, -1.000000000000000000 ) ) ;
#16149=EDGE_CURVE ( 'NONE', #25123, #20874, #21051, .T. ) ;
#16169=CARTESIAN_POINT ( 'NONE',  ( -305.0000000000001137, -170.0000000000001137, 60.00000000000002842 ) ) ;
#16178=EDGE_CURVE ( 'NONE', #27270, #3147, #2074, .T. ) ;
#16212=VECTOR ( 'NONE', #288, 1000.000000000000000 ) ;
#16226=CARTESIAN_POINT ( 'NONE',  ( -210.0000000000000568, -213.8933171992501059, 90.09368185681027796 ) ) ;
#16233=CARTESIAN_POINT ( 'NONE',  ( -212.2419371577844345, -220.0000000000000853, -110.0000000000000284 ) ) ;
#16240=ORIENTED_EDGE ( 'NONE', *, *, #18193, .F. ) ;
#16266=DIRECTION ( 'NONE',  ( -2.775557561562887407E-16, -3.668437989309015850E-32, 1.000000000000000000 ) ) ;
#16299=VECTOR ( 'NONE', #25768, 1000.000000000000000 ) ;
#16309=ORIENTED_EDGE ( 'NONE', *, *, #6502, .F. ) ;
#16311=EDGE_CURVE ( 'NONE', #24757, #28358, #14654, .T. ) ;
#16349=DIRECTION ( 'NONE',  ( 0.9711705445023437466, -0.2383857661250380899, 0.000000000000000000 ) ) ;
#16350=EDGE_LOOP ( 'NONE', ( #10789, #18103, #8311, #26006 ) ) ;
#16352=LINE ( 'NONE', #13775, #12781 ) ;
#16469=EDGE_CURVE ( 'NONE', #10091, #17968, #19225, .T. ) ;
#16476=CIRCLE ( 'NONE', #3142, 67.21503689626328537 ) ;
#16494=CARTESIAN_POINT ( 'NONE',  ( -212.2419371577844345, -220.0000000000000853, -94.99999999999987210 ) ) ;
#16506=CARTESIAN_POINT ( 'NONE',  ( -268.8075929731044766, -170.5243996965605504, -94.03848302756206579 ) ) ;
#16507=DIRECTION ( 'NONE',  ( -0.000000000000000000, -1.000000000000000000, -0.000000000000000000 ) ) ;
#16601=CARTESIAN_POINT ( 'NONE',  ( -305.0000000000001137, -170.0000000000001137, -59.99999999999986500 ) ) ;
#16606=VECTOR ( 'NONE', #20311, 1000.000000000000000 ) ;
#16609=CARTESIAN_POINT ( 'NONE',  ( -210.0000000000000568, -220.0000000000000853, 90.87829376371914236 ) ) ;
#16626=EDGE_CURVE ( 'NONE', #5554, #27204, #16930, .T. ) ;
#16632=AXIS2_PLACEMENT_3D ( 'NONE', #586, #9352, #3144 ) ;
#16661=EDGE_CURVE ( 'NONE', #21378, #22270, #22850, .T. ) ;
#16685=DIRECTION ( 'NONE',  ( -0.2383857661250380344, -0.9711705445023436356, 0.000000000000000000 ) ) ;
#16704=DIRECTION ( 'NONE',  ( -4.625929269271489858E-16, 2.100614451407711032E-31, -1.000000000000000000 ) ) ;
#16709=DIRECTION ( 'NONE',  ( 1.000000000000000000, 1.321694076934710155E-16, -0.000000000000000000 ) ) ;
#16741=CARTESIAN_POINT ( 'NONE',  ( -210.0000000000000853, -213.8933171992502196, 109.9063181431897505 ) ) ;
#16779=CARTESIAN_POINT ( 'NONE',  ( -270.9384205528269831, -170.2669023585998218, 87.94298069144645069 ) ) ;
#16800=VERTEX_POINT ( 'NONE', #9226 ) ;
#16856=EDGE_LOOP ( 'NONE', ( #23975, #15867, #9109, #11793 ) ) ;
#16869=ORIENTED_EDGE ( 'NONE', *, *, #16626, .F. ) ;
#16886=ORIENTED_EDGE ( 'NONE', *, *, #24445, .F. ) ;
#16906=ORIENTED_EDGE ( 'NONE', *, *, #17610, .T. ) ;
#16930=CIRCLE ( 'NONE', #8210, 49.99999999999998579 ) ;
#17010=CARTESIAN_POINT ( 'NONE',  ( -277.2150368962633706, -237.2150368962634559, 110.0000000000000142 ) ) ;
#17012=CARTESIAN_POINT ( 'NONE',  ( -210.0000000000000568, -210.8114316696540982, 110.0000000000000284 ) ) ;
#17018=ORIENTED_EDGE ( 'NONE', *, *, #8675, .F. ) ;
#17029=DIRECTION ( 'NONE',  ( 4.540956701092242152E-16, 1.000000000000000000, 0.000000000000000000 ) ) ;
#17030=CARTESIAN_POINT ( 'NONE',  ( -210.0000000000001137, -157.0000000000000284, 105.0000000000000284 ) ) ;
#17051=CIRCLE ( 'NONE', #11087, 67.21503689626328537 ) ;
#17071=ORIENTED_EDGE ( 'NONE', *, *, #8675, .T. ) ;
#17075=VERTEX_POINT ( 'NONE', #13461 ) ;
#17093=CYLINDRICAL_SURFACE ( 'NONE', #18290, 5.000000000000004441 ) ;
#17098=VERTEX_POINT ( 'NONE', #19767 ) ;
#17101=CARTESIAN_POINT ( 'NONE',  ( -264.1793819498149674, -171.2044657688920211, -109.9235875798455027 ) ) ;
#17118=EDGE_LOOP ( 'NONE', ( #15332, #7404, #23653, #17018, #6343, #5971 ) ) ;
#17125=CARTESIAN_POINT ( 'NONE',  ( -260.0000000000001137, -167.0819201924624906, -89.99999999999985789 ) ) ;
#17134=ORIENTED_EDGE ( 'NONE', *, *, #5146, .T. ) ;
#17185=CARTESIAN_POINT ( 'NONE',  ( -210.0000000000000568, -210.8114316696540982, -110.0000000000000284 ) ) ;
#17200=DIRECTION ( 'NONE',  ( 0.000000000000000000, 0.000000000000000000, -1.000000000000000000 ) ) ;
#17206=DIRECTION ( 'NONE',  ( -0.4918581970360879074, 0.000000000000000000, -0.8706753206611571594 ) ) ;
#17219=ORIENTED_EDGE ( 'NONE', *, *, #5982, .F. ) ;
#17229=B_SPLINE_CURVE_WITH_KNOTS ( 'NONE', 3,
 ( #21504, #1821, #10596, #23107, #1263, #28100, #16506, #14349, #17623, #15344, #19918, #4680 ),
 .UNSPECIFIED., .F., .F.,
 ( 4, 2, 2, 2, 2, 4 ),
 ( 0.000000000000000000, 0.004258390697697790085, 0.006387586046546603162, 0.008516781395395417106, 0.01277517209309319245, 0.01703356279079096952 ),
 .UNSPECIFIED. ) ;
#17230=DIRECTION ( 'NONE',  ( 1.000000000000000000, 0.000000000000000000, 0.000000000000000000 ) ) ;
#17234=FACE_OUTER_BOUND ( 'NONE', #25236, .T. ) ;
#17240=CARTESIAN_POINT ( 'NONE',  ( -267.2062018704829143, -170.6788222641287120, -109.5782777413358389 ) ) ;
#17288=ORIENTED_EDGE ( 'NONE', *, *, #6323, .T. ) ;
#17332=CARTESIAN_POINT ( 'NONE',  ( -268.0371306804030951, -170.6155949349647756, 94.25159887050631369 ) ) ;
#17342=AXIS2_PLACEMENT_3D ( 'NONE', #10665, #8933, #19425 ) ;
#17370=VECTOR ( 'NONE', #10426, 1000.000000000000000 ) ;
#17378=VECTOR ( 'NONE', #6175, 1000.000000000000000 ) ;
#17381=CARTESIAN_POINT ( 'NONE',  ( -263.2300671076336016, -166.3683464297101580, -109.9999999999998721 ) ) ;
#17407=EDGE_LOOP ( 'NONE', ( #6814, #13412, #14304, #15855 ) ) ;
#17410=DIRECTION ( 'NONE',  ( 5.551115123125777969E-15, 0.000000000000000000, 1.000000000000000000 ) ) ;
#17449=CARTESIAN_POINT ( 'NONE',  ( -273.6135038633245244, -165.0000000000001705, 86.76553013670502423 ) ) ;
#17450=CARTESIAN_POINT ( 'NONE',  ( -277.2150368962633706, -237.2150368962634559, 105.0000000000000000 ) ) ;
#17468=CARTESIAN_POINT ( 'NONE',  ( -213.1827219047386848, -216.7767438708612531, 95.00000000000004263 ) ) ;
#17471=CARTESIAN_POINT ( 'NONE',  ( -260.0000000000001137, -157.0000000000000284, 110.0000000000000142 ) ) ;
#17523=ADVANCED_FACE ( 'NONE', ( #25809 ), #12134, .T. ) ;
#17531=B_SPLINE_CURVE_WITH_KNOTS ( 'NONE', 3,
 ( #15897, #22639, #6965, #9563, #11440, #932, #515, #2798 ),
 .UNSPECIFIED., .F., .F.,
 ( 4, 2, 2, 4 ),
 ( 0.000000000000000000, 0.004190943542067912184, 0.008381887084135824367, 0.01676377416827165567 ),
 .UNSPECIFIED. ) ;
#17539=CARTESIAN_POINT ( 'NONE',  ( -210.8169819562698137, -219.6631312228495858, 108.5590195769788551 ) ) ;
#17552=CARTESIAN_POINT ( 'NONE',  ( -211.4344004814429923, -220.0000000000001137, -107.6907272673696383 ) ) ;
#17563=LINE ( 'NONE', #23896, #23020 ) ;
#17570=ORIENTED_EDGE ( 'NONE', *, *, #24100, .T. ) ;
#17586=DIRECTION ( 'NONE',  ( -1.321694076934710155E-16, 1.000000000000000000, 0.000000000000000000 ) ) ;
#17610=EDGE_CURVE ( 'NONE', #13525, #22223, #6983, .T. ) ;
#17622=B_SPLINE_CURVE_WITH_KNOTS ( 'NONE', 3,
 ( #17012, #5534, #16741, #3513, #21039, #19030 ),
 .UNSPECIFIED., .F., .F.,
 ( 4, 2, 4 ),
 ( 0.000000000000000000, 0.004615224477119856880, 0.009230448954239713760 ),
 .UNSPECIFIED. ) ;
#17623=CARTESIAN_POINT ( 'NONE',  ( -272.1612352632698162, -170.1778405466225763, -92.98998843785479096 ) ) ;
#17660=CARTESIAN_POINT ( 'NONE',  ( -260.0000000000001137, -165.0000000000001137, -59.99999999999986500 ) ) ;
#17676=AXIS2_PLACEMENT_3D ( 'NONE', #245, #26507, #17757 ) ;
#17683=CIRCLE ( 'NONE', #721, 4.999999999999992895 ) ;
#17757=DIRECTION ( 'NONE',  ( -1.000000000000000000, 4.540956701092242152E-16, 0.000000000000000000 ) ) ;
#17774=( NAMED_UNIT ( * ) PLANE_ANGLE_UNIT ( ) SI_UNIT ( $, .RADIAN. ) );
#17796=CARTESIAN_POINT ( 'NONE',  ( -260.0000000000001137, -165.0000000000001137, 60.00000000000002132 ) ) ;
#17799=DIRECTION ( 'NONE',  ( 4.540956701092242152E-16, 1.000000000000000000, 0.000000000000000000 ) ) ;
#17836=FACE_OUTER_BOUND ( 'NONE', #1567, .T. ) ;
#17851=CIRCLE ( 'NONE', #8688, 67.21503689626328537 ) ;
#17854=VECTOR ( 'NONE', #23534, 1000.000000000000000 ) ;
#17860=EDGE_CURVE ( 'NONE', #4420, #4251, #1368, .T. ) ;
#17865=CARTESIAN_POINT ( 'NONE',  ( -274.6583047828685835, -170.0000000000001137, 102.7143168399017270 ) ) ;
#17905=DIRECTION ( 'NONE',  ( 1.000000000000000000, 0.000000000000000000, 0.000000000000000000 ) ) ;
#17968=VERTEX_POINT ( 'NONE', #8547 ) ;
#17973=CARTESIAN_POINT ( 'NONE',  ( -210.0000000000000568, -220.0000000000000853, 109.1217062362809145 ) ) ;
#17990=CARTESIAN_POINT ( 'NONE',  ( -260.0000000000001137, -157.0000000000000284, -89.99999999999985789 ) ) ;
#18045=ORIENTED_EDGE ( 'NONE', *, *, #25057, .F. ) ;
#18052=EDGE_CURVE ( 'NONE', #3368, #25077, #26720, .T. ) ;
#18070=AXIS2_PLACEMENT_3D ( 'NONE', #12137, #11852, #9687 ) ;
#18101=CARTESIAN_POINT ( 'NONE',  ( -260.0000000000001137, -157.0000000000000284, 95.00000000000001421 ) ) ;
#18103=ORIENTED_EDGE ( 'NONE', *, *, #24536, .F. ) ;
#18155=PLANE ( 'NONE',  #25026 ) ;
#18193=EDGE_CURVE ( 'NONE', #12640, #5842, #25351, .T. ) ;
#18214=VERTEX_POINT ( 'NONE', #1743 ) ;
#18290=AXIS2_PLACEMENT_3D ( 'NONE', #1715, #8904, #28137 ) ;
#18296=VECTOR ( 'NONE', #7138, 1000.000000000000000 ) ;
#18347=LINE ( 'NONE', #15774, #18296 ) ;
#18378=DIRECTION ( 'NONE',  ( 4.540956701092242152E-16, 1.000000000000000000, 0.000000000000000000 ) ) ;
#18390=FACE_OUTER_BOUND ( 'NONE', #2463, .T. ) ;
#18491=EDGE_LOOP ( 'NONE', ( #4593, #3430, #23478, #11598 ) ) ;
#18493=CIRCLE ( 'NONE', #12984, 5.000000000000004441 ) ;
#18522=ADVANCED_FACE ( 'NONE', ( #7738 ), #974, .T. ) ;
#18552=ORIENTED_EDGE ( 'NONE', *, *, #9628, .T. ) ;
#18556=ORIENTED_EDGE ( 'NONE', *, *, #5477, .F. ) ;
#18571=DIRECTION ( 'NONE',  ( -1.321694076934710155E-16, 1.000000000000000000, 0.000000000000000000 ) ) ;
#18595=EDGE_CURVE ( 'NONE', #21378, #21916, #1264, .T. ) ;
#18603=EDGE_CURVE ( 'NONE', #25748, #3224, #2351, .T. ) ;
#18607=CIRCLE ( 'NONE', #22277, 5.000000000000004441 ) ;
#18635=AXIS2_PLACEMENT_3D ( 'NONE', #25458, #9819, #23307 ) ;
#18642=CARTESIAN_POINT ( 'NONE',  ( -211.0641392867345871, -220.0000000000001137, -91.81659942089190451 ) ) ;
#18685=CARTESIAN_POINT ( 'NONE',  ( -277.2150368962633706, -237.2150368962634559, 105.0000000000000000 ) ) ;
#18704=CARTESIAN_POINT ( 'NONE',  ( -210.0000000000000568, -220.0000000000000853, -90.87829376371895762 ) ) ;
#18712=FACE_OUTER_BOUND ( 'NONE', #23718, .T. ) ;
#18756=DIRECTION ( 'NONE',  ( -1.000000000000000000, 0.000000000000000000, 0.000000000000000000 ) ) ;
#18781=CARTESIAN_POINT ( 'NONE',  ( -210.3420575078734771, -220.0000000000000284, -91.10584728836482782 ) ) ;
#18800=ORIENTED_EDGE ( 'NONE', *, *, #6731, .F. ) ;
#18801=AXIS2_PLACEMENT_3D ( 'NONE', #24953, #821, #22225 ) ;
#18809=ORIENTED_EDGE ( 'NONE', *, *, #9496, .F. ) ;
#18845=CARTESIAN_POINT ( 'NONE',  ( -277.2150368962633706, -237.2150368962634559, -94.99999999999985789 ) ) ;
#18861=CARTESIAN_POINT ( 'NONE',  ( -210.0000000000000568, -157.0000000000000284, -110.0000000000000284 ) ) ;
#18875=ORIENTED_EDGE ( 'NONE', *, *, #24097, .T. ) ;
#18885=ADVANCED_FACE ( 'NONE', ( #9151 ), #19832, .T. ) ;
#18918=VERTEX_POINT ( 'NONE', #16609 ) ;
#18920=CYLINDRICAL_SURFACE ( 'NONE', #11813, 49.99999999999998579 ) ;
#18924=CIRCLE ( 'NONE', #3781, 5.000000000000004441 ) ;
#18930=CARTESIAN_POINT ( 'NONE',  ( -270.6423355020924646, -165.1562042664794774, 88.05640019106880345 ) ) ;
#18933=DIRECTION ( 'NONE',  ( -1.000000000000000000, 0.000000000000000000, 3.074769666655405408E-15 ) ) ;
#18946=ORIENTED_EDGE ( 'NONE', *, *, #22268, .T. ) ;
#18996=LINE ( 'NONE', #25320, #26879 ) ;
#18998=DIRECTION ( 'NONE',  ( 1.000000000000000000, 0.000000000000000000, 0.000000000000000000 ) ) ;
#19024=ORIENTED_EDGE ( 'NONE', *, *, #26101, .T. ) ;
#19030=CARTESIAN_POINT ( 'NONE',  ( -210.0000000000000568, -220.0000000000000853, 109.1217062362809145 ) ) ;
#19059=ORIENTED_EDGE ( 'NONE', *, *, #14231, .T. ) ;
#19067=CARTESIAN_POINT ( 'NONE',  ( -265.0761585189258653, -165.8845232629588793, -89.57447787032170083 ) ) ;
#19155=CARTESIAN_POINT ( 'NONE',  ( -213.1827219047386848, -216.7767438708612531, 95.00000000000004263 ) ) ;
#19218=ORIENTED_EDGE ( 'NONE', *, *, #27847, .T. ) ;
#19225=CIRCLE ( 'NONE', #13750, 72.21503689626329958 ) ;
#19232=ORIENTED_EDGE ( 'NONE', *, *, #16661, .F. ) ;
#19292=DIRECTION ( 'NONE',  ( 0.000000000000000000, 0.000000000000000000, 1.000000000000000000 ) ) ;
#19304=AXIS2_PLACEMENT_3D ( 'NONE', #984, #16507, #20809 ) ;
#19325=CARTESIAN_POINT ( 'NONE',  ( -268.1539709403929805, -165.4081636382954343, 88.87781807846162963 ) ) ;
#19327=DIRECTION ( 'NONE',  ( 4.540956701092242152E-16, 1.000000000000000000, 0.000000000000000000 ) ) ;
#19347=CARTESIAN_POINT ( 'NONE',  ( -265.2785062999343495, -171.0615922813920804, -89.54987397248345360 ) ) ;
#19348=CARTESIAN_POINT ( 'NONE',  ( -270.7452880837828388, -170.3087097900280753, 93.46977427553774476 ) ) ;
#19350=EDGE_CURVE ( 'NONE', #8779, #28324, #5365, .T. ) ;
#19368=B_SPLINE_CURVE_WITH_KNOTS ( 'NONE', 3,
 ( #27809, #4255, #8147, #25806, #6132, #13042, #23801, #10735, #6414, #15191, #28364, #23943, #21789, #2096, #8714, #17468 ),
 .UNSPECIFIED., .F., .F.,
 ( 4, 2, 2, 2, 2, 2, 2, 4 ),
 ( 0.000000000000000000, 0.001557302553632627148, 0.002335953830448963056, 0.003114605107265298531, 0.004671907660897984226, 0.005450558937714350925, 0.005839884576122509122, 0.006229210214530666451 ),
 .UNSPECIFIED. ) ;
#19384=DIRECTION ( 'NONE',  ( 1.000000000000000000, 1.321694076934710155E-16, 0.000000000000000000 ) ) ;
#19406=ORIENTED_EDGE ( 'NONE', *, *, #10014, .F. ) ;
#19411=CIRCLE ( 'NONE', #10701, 5.000000000000004441 ) ;
#19413=PLANE ( 'NONE',  #24744 ) ;
#19417=CARTESIAN_POINT ( 'NONE',  ( -295.0000000000001705, -165.0000000000001137, -110.0000000000000426 ) ) ;
#19418=B_SPLINE_CURVE_WITH_KNOTS ( 'NONE', 3,
 ( #10025, #18781, #20795, #18642, #27387, #11913, #973, #25527, #7593, #7861, #5847, #7728, #16494 ),
 .UNSPECIFIED., .F., .F.,
 ( 4, 2, 2, 1, 2, 2, 4 ),
 ( 0.000000000000000000, 0.001215484442346315792, 0.001823226663519458618, 0.002430968884692601226, 0.003038711105865744052, 0.003646453327038886878, 0.004861937769385192044 ),
 .UNSPECIFIED. ) ;
#19425=DIRECTION ( 'NONE',  ( -1.000000000000000000, 0.000000000000000000, 0.000000000000000000 ) ) ;
#19464=ORIENTED_EDGE ( 'NONE', *, *, #9256, .T. ) ;
#19494=CARTESIAN_POINT ( 'NONE',  ( -261.1919288306253293, -171.9377729149742038, -94.99999999999987210 ) ) ;
#19495=CARTESIAN_POINT ( 'NONE',  ( -265.0505472617491023, -165.8775750992075189, 89.59901895717871412 ) ) ;
#19510=CIRCLE ( 'NONE', #8963, 35.00000000000000711 ) ;
#19513=ORIENTED_EDGE ( 'NONE', *, *, #16311, .F. ) ;
#19560=CARTESIAN_POINT ( 'NONE',  ( -211.7958164186347290, -218.9496041985362922, 107.5698157934932766 ) ) ;
#19575=CARTESIAN_POINT ( 'NONE',  ( -212.2419371577844345, -220.0000000000000853, -105.0000000000000284 ) ) ;
#19584=ADVANCED_FACE ( 'NONE', ( #17836 ), #175, .T. ) ;
#19618=CARTESIAN_POINT ( 'NONE',  ( -266.7059280454142822, -170.8119893264861844, 94.52701477642899874 ) ) ;
#19623=EDGE_CURVE ( 'NONE', #5842, #4420, #12958, .T. ) ;
#19655=AXIS2_PLACEMENT_3D ( 'NONE', #17030, #12035, #23082 ) ;
#19662=ADVANCED_FACE ( 'NONE', ( #15552 ), #24302, .T. ) ;
#19700=CARTESIAN_POINT ( 'NONE',  ( -213.1553235149991110, -216.8625818769947955, 105.0933958169749047 ) ) ;
#19744=VERTEX_POINT ( 'NONE', #11538 ) ;
#19754=CARTESIAN_POINT ( 'NONE',  ( -272.1218244932625225, -170.1898742340911781, 92.97996575210989079 ) ) ;
#19767=CARTESIAN_POINT ( 'NONE',  ( -305.0000000000001137, -170.0000000000001137, -59.99999999999987210 ) ) ;
#19780=EDGE_CURVE ( 'NONE', #268, #22186, #2857, .T. ) ;
#19786=ORIENTED_EDGE ( 'NONE', *, *, #12227, .T. ) ;
#19832=( BOUNDED_SURFACE ( )  B_SPLINE_SURFACE ( 3, 2, ( 
 ( #9999, #5116, #25365 ),
 ( #20912, #20349, #22656 ),
 ( #14315, #27094, #2815 ),
 ( #817, #3095, #14047 ),
 ( #12024, #5541, #12169 ),
 ( #9721, #3236, #27505 ),
 ( #681, #13908, #24807 ),
 ( #2963, #11753, #20769 ) ),
 .UNSPECIFIED., .F., .F., .F. ) 
 B_SPLINE_SURFACE_WITH_KNOTS ( ( 4, 2, 2, 4 ),
 ( 3, 3 ),
 ( 0.000000000000000000, 0.008853367702742013026, 0.01328005155411302041, 0.01770673540548402605 ),
 ( 0.000000000000000000, 1.000000000000000000 ),
 .UNSPECIFIED. ) 
 GEOMETRIC_REPRESENTATION_ITEM ( )  RATIONAL_B_SPLINE_SURFACE ( (
 ( 1.000000000000000000, 0.7071067811865475727, 1.000000000000000000),
 ( 1.000000000000000000, 0.7122833902602503375, 1.000000000000000000),
 ( 1.000000000000000000, 0.7150365851228822622, 1.000000000000000000),
 ( 1.000000000000000000, 0.7151618057631559111, 1.000000000000000000),
 ( 1.000000000000000000, 0.7145339593740676065, 1.000000000000000000),
 ( 1.000000000000000000, 0.7118598333332957218, 1.000000000000000000),
 ( 1.000000000000000000, 0.7098294805783303962, 1.000000000000000000),
 ( 1.000000000000000000, 0.7071067811865465735, 1.000000000000000000) ) ) 
 REPRESENTATION_ITEM ( '' )  SURFACE ( )  );
#19840=CARTESIAN_POINT ( 'NONE',  ( -260.0000000000001137, -152.0000000000000284, -104.9999999999998721 ) ) ;
#19875=CIRCLE ( 'NONE', #12086, 30.00000000000000711 ) ;
#19894=CARTESIAN_POINT ( 'NONE',  ( -260.0000000000001137, -170.0000000000001137, -59.99999999999986500 ) ) ;
#19913=ADVANCED_FACE ( 'NONE', ( #3448 ), #26253, .T. ) ;
#19915=FACE_OUTER_BOUND ( 'NONE', #10381, .T. ) ;
#19918=CARTESIAN_POINT ( 'NONE',  ( -275.9937304809269563, -170.0000000000001421, -91.21489442788019630 ) ) ;
#19923=ORIENTED_EDGE ( 'NONE', *, *, #2019, .F. ) ;
#19946=CARTESIAN_POINT ( 'NONE',  ( -277.2150368962633706, -237.2150368962634559, -110.0000000000000284 ) ) ;
#19974=ORIENTED_EDGE ( 'NONE', *, *, #400, .T. ) ;
#20051=CLOSED_SHELL ( 'NONE', ( #21834, #1810, #14290, #173, #11742, #9565, #6818, #3931, #19662, #27565, #473, #7023, #2634, #4503, #1993, #23028, #26539, #7933, #13948, #13171, #2566, #2494, #18885, #12619, #539, #7293, #2453, #4594, #22398, #5775, #17523, #19913, #10612, #13393, #3995, #4546, #15944, #28010, #18522, #8665, #21088, #19584 ) ) ;
#20053=DIRECTION ( 'NONE',  ( 0.000000000000000000, 0.000000000000000000, 1.000000000000000000 ) ) ;
#20063=EDGE_CURVE ( 'NONE', #25077, #28289, #21683, .T. ) ;
#20113=DIRECTION ( 'NONE',  ( 0.000000000000000000, 0.000000000000000000, -1.000000000000000000 ) ) ;
#20146=MECHANICAL_DESIGN_GEOMETRIC_PRESENTATION_REPRESENTATION('',(#2715),#7324);
#20192=EDGE_CURVE ( 'NONE', #25123, #23090, #18493, .T. ) ;
#20201=CARTESIAN_POINT ( 'NONE',  ( -305.0000000000001137, -165.0000000000001137, -110.0000000000000284 ) ) ;
#20222=ORIENTED_EDGE ( 'NONE', *, *, #12953, .F. ) ;
#20233=DIRECTION ( 'NONE',  ( 0.000000000000000000, -0.000000000000000000, 1.000000000000000000 ) ) ;
#20256=CYLINDRICAL_SURFACE ( 'NONE', #16632, 5.000000000000004441 ) ;
#20301=FACE_OUTER_BOUND ( 'NONE', #9705, .T. ) ;
#20311=DIRECTION ( 'NONE',  ( -4.625929269271489858E-16, 0.000000000000000000, -1.000000000000000000 ) ) ;
#20324=CARTESIAN_POINT ( 'NONE',  ( -260.0000000000001137, -152.0000000000000284, 60.00000000000002132 ) ) ;
#20349=CARTESIAN_POINT ( 'NONE',  ( -276.2395898676904835, -169.9272804698039749, 107.3924858170726964 ) ) ;
#20418=CARTESIAN_POINT ( 'NONE',  ( -274.7557459110829541, -165.0000000000001137, -86.12025961983451339 ) ) ;
#20439=CARTESIAN_POINT ( 'NONE',  ( -210.0000000000000568, -216.9546086794800317, -90.40281535134946012 ) ) ;
#20450=AXIS2_PLACEMENT_3D ( 'NONE', #24803, #15912, #5257 ) ;
#20477=ORIENTED_EDGE ( 'NONE', *, *, #28050, .F. ) ;
#20520=CARTESIAN_POINT ( 'NONE',  ( -210.0000000000000568, -220.0000000000000853, 90.87829376371914236 ) ) ;
#20556=CARTESIAN_POINT ( 'NONE',  ( -305.0000000000001137, -157.0000000000000284, -59.99999999999987210 ) ) ;
#20590=CARTESIAN_POINT ( 'NONE',  ( -265.0574300291106056, -165.8879864452689219, -89.57768297750722297 ) ) ;
#20609=CIRCLE ( 'NONE', #26115, 44.99999999999999289 ) ;
#20623=B_SPLINE_CURVE_WITH_KNOTS ( 'NONE', 3,
 ( #1181, #27181, #23159, #20439, #9947, #18704 ),
 .UNSPECIFIED., .F., .F.,
 ( 4, 2, 4 ),
 ( 0.000000000000000000, 0.004615224477119856880, 0.009230448954239713760 ),
 .UNSPECIFIED. ) ;
#20624=AXIS2_PLACEMENT_3D ( 'NONE', #9811, #18571, #27316 ) ;
#20644=DIRECTION ( 'NONE',  ( -1.000000000000000000, 0.000000000000000000, 0.000000000000000000 ) ) ;
#20649=ORIENTED_EDGE ( 'NONE', *, *, #22490, .F. ) ;
#20657=DIRECTION ( 'NONE',  ( -0.000000000000000000, -1.000000000000000000, -0.000000000000000000 ) ) ;
#20718=AXIS2_PLACEMENT_3D ( 'NONE', #6927, #187, #15288 ) ;
#20729=ORIENTED_EDGE ( 'NONE', *, *, #20943, .F. ) ;
#20738=CARTESIAN_POINT ( 'NONE',  ( -295.0000000000001137, -170.0000000000001137, 60.00000000000002842 ) ) ;
#20762=EDGE_CURVE ( 'NONE', #24423, #21378, #17051, .T. ) ;
#20769=CARTESIAN_POINT ( 'NONE',  ( -260.0000000000001705, -167.0819201924624622, 110.0000000000000142 ) ) ;
#20783=ORIENTED_EDGE ( 'NONE', *, *, #3451, .F. ) ;
#20795=CARTESIAN_POINT ( 'NONE',  ( -210.6507024897083795, -220.0000000000000853, -91.36902465222451042 ) ) ;
#20809=DIRECTION ( 'NONE',  ( 0.000000000000000000, 0.000000000000000000, -1.000000000000000000 ) ) ;
#20826=ORIENTED_EDGE ( 'NONE', *, *, #15521, .F. ) ;
#20855=AXIS2_PLACEMENT_3D ( 'NONE', #12657, #19384, #25845 ) ;
#20857=DIRECTION ( 'NONE',  ( 0.000000000000000000, 0.000000000000000000, -1.000000000000000000 ) ) ;
#20874=VERTEX_POINT ( 'NONE', #6775 ) ;
#20883=ORIENTED_EDGE ( 'NONE', *, *, #27961, .F. ) ;
#20912=CARTESIAN_POINT ( 'NONE',  ( -274.6409284829297803, -170.0000000000001421, 102.7220467394344894 ) ) ;
#20924=CARTESIAN_POINT ( 'NONE',  ( -260.0000000000001137, -220.0000000000000853, -59.99999999999986500 ) ) ;
#20934=DIRECTION ( 'NONE',  ( -1.321694076934710155E-16, 1.000000000000000000, 0.000000000000000000 ) ) ;
#20943=EDGE_CURVE ( 'NONE', #4251, #6860, #9229, .T. ) ;
#20996=CARTESIAN_POINT ( 'NONE',  ( -277.2150368962633706, -165.0000000000001137, 101.5769467933889416 ) ) ;
#20998=DIRECTION ( 'NONE',  ( -1.000000000000000000, 0.000000000000000000, 0.000000000000000000 ) ) ;
#20999=DIRECTION ( 'NONE',  ( -1.000000000000000000, 6.167905692361982533E-16, 0.000000000000000000 ) ) ;
#21036=ORIENTED_EDGE ( 'NONE', *, *, #13251, .T. ) ;
#21039=CARTESIAN_POINT ( 'NONE',  ( -210.0000000000000853, -218.4793454996984394, 109.3807997302053963 ) ) ;
#21051=LINE ( 'NONE', #1655, #17370 ) ;
#21079=CARTESIAN_POINT ( 'NONE',  ( -265.8568188415123359, -170.9585686148244292, -89.43929063625722620 ) ) ;
#21080=CARTESIAN_POINT ( 'NONE',  ( -210.0000000000000853, -212.3568517473289603, 90.00000000000004263 ) ) ;
#21087=VERTEX_POINT ( 'NONE', #978 ) ;
#21088=ADVANCED_FACE ( 'NONE', ( #11917 ), #23105, .T. ) ;
#21112=CARTESIAN_POINT ( 'NONE',  ( -276.0340605539078638, -165.0395234928621448, -107.3883478461701912 ) ) ;
#21122=CARTESIAN_POINT ( 'NONE',  ( -279.1278187736259611, -165.0000000000001137, -106.1966075482098262 ) ) ;
#21133=ORIENTED_EDGE ( 'NONE', *, *, #21742, .F. ) ;
#21219=CARTESIAN_POINT ( 'NONE',  ( -268.0810832944869162, -170.6198684656366140, -94.21671656981227727 ) ) ;
#21232=CARTESIAN_POINT ( 'NONE',  ( -277.2150368962633706, -165.0000000000001421, -101.5769467933887995 ) ) ;
#21252=DIRECTION ( 'NONE',  ( -1.321694076934710155E-16, 1.000000000000000000, 0.000000000000000000 ) ) ;
#21266=CARTESIAN_POINT ( 'NONE',  ( -276.0275629839314320, -165.0396948272157829, -107.3906533568332122 ) ) ;
#21272=ORIENTED_EDGE ( 'NONE', *, *, #22635, .F. ) ;
#21289=FACE_OUTER_BOUND ( 'NONE', #7558, .T. ) ;
#21378=VERTEX_POINT ( 'NONE', #3325 ) ;
#21432=CARTESIAN_POINT ( 'NONE',  ( -310.0000000000001137, -165.0000000000001137, 60.00000000000001421 ) ) ;
#21437=DIRECTION ( 'NONE',  ( -1.000000000000000000, 0.000000000000000000, 0.000000000000000000 ) ) ;
#21459=CIRCLE ( 'NONE', #17342, 5.000000000000004441 ) ;
#21475=CIRCLE ( 'NONE', #11865, 5.000000000000004441 ) ;
#21498=CARTESIAN_POINT ( 'NONE',  ( -268.7670636128347041, -170.5295276737763857, -94.04889937631023145 ) ) ;
#21500=CARTESIAN_POINT ( 'NONE',  ( -266.6762645635436115, -170.8168138549905279, 94.53218878333569819 ) ) ;
#21504=CARTESIAN_POINT ( 'NONE',  ( -261.1919288306253293, -171.9377729149742038, -94.99999999999987210 ) ) ;
#21536=CARTESIAN_POINT ( 'NONE',  ( -263.2410596828399889, -166.3659179929189236, -109.9999999999998863 ) ) ;
#21544=CARTESIAN_POINT ( 'NONE',  ( -310.0000000000001137, -165.0000000000000853, 60.00000000000002842 ) ) ;
#21550=CARTESIAN_POINT ( 'NONE',  ( -274.6179956896274916, -170.0369464504329926, -102.6515880211471199 ) ) ;
#21552=PRODUCT_CONTEXT ( 'NONE', #15356, 'mechanical' ) ;
#21588=ORIENTED_EDGE ( 'NONE', *, *, #10014, .T. ) ;
#21621=CARTESIAN_POINT ( 'NONE',  ( -274.7557459110829541, -165.0000000000001421, 86.12025961983462707 ) ) ;
#21646=VECTOR ( 'NONE', #12741, 1000.000000000000000 ) ;
#21647=CARTESIAN_POINT ( 'NONE',  ( -274.7130711414566235, -170.0340489564030690, -91.87824641412829862 ) ) ;
#21648=CARTESIAN_POINT ( 'NONE',  ( -272.0864800775726167, -170.1925618487048268, 92.99347412766374532 ) ) ;
#21676=EDGE_CURVE ( 'NONE', #2951, #21916, #19418, .T. ) ;
#21683=CIRCLE ( 'NONE', #594, 44.99999999999998579 ) ;
#21701=AXIS2_PLACEMENT_3D ( 'NONE', #17010, #23342, #10550 ) ;
#21738=VERTEX_POINT ( 'NONE', #22817 ) ;
#21742=EDGE_CURVE ( 'NONE', #22223, #18214, #8843, .T. ) ;
#21789=CARTESIAN_POINT ( 'NONE',  ( -213.0597602322721116, -217.1208202143830590, 94.62152100247507747 ) ) ;
#21834=ADVANCED_FACE ( 'NONE', ( #28233 ), #1812, .T. ) ;
#21838=CARTESIAN_POINT ( 'NONE',  ( -277.2150368962633706, -237.2150368962634559, -104.9999999999998153 ) ) ;
#21846=EDGE_CURVE ( 'NONE', #18918, #10018, #19368, .T. ) ;
#21860=CARTESIAN_POINT ( 'NONE',  ( -213.0248109774373972, -217.2055523511229467, 105.4731297167887902 ) ) ;
#21916=VERTEX_POINT ( 'NONE', #5387 ) ;
#21921=ORIENTED_EDGE ( 'NONE', *, *, #27879, .F. ) ;
#21937=DIRECTION ( 'NONE',  ( 0.000000000000000000, 0.000000000000000000, -1.000000000000000000 ) ) ;
#21972=ORIENTED_EDGE ( 'NONE', *, *, #28050, .T. ) ;
#21999=EDGE_LOOP ( 'NONE', ( #17288, #3884, #20826, #7476 ) ) ;
#22011=ORIENTED_EDGE ( 'NONE', *, *, #22490, .T. ) ;
#22012=( NAMED_UNIT ( * ) SI_UNIT ( $, .STERADIAN. ) SOLID_ANGLE_UNIT ( ) );
#22027=EDGE_CURVE ( 'NONE', #3702, #9462, #22150, .T. ) ;
#22034=CARTESIAN_POINT ( 'NONE',  ( -263.9162289044071485, -171.3140465951013311, 104.9290552840942325 ) ) ;
#22040=DIRECTION ( 'NONE',  ( 0.000000000000000000, 0.000000000000000000, -1.000000000000000000 ) ) ;
#22052=ORIENTED_EDGE ( 'NONE', *, *, #19623, .T. ) ;
#22061=B_SPLINE_CURVE_WITH_KNOTS ( 'NONE', 3,
 ( #17973, #13115, #17539, #10804, #11231, #19560, #164, #24292, #13386, #13533, #28301, #21860, #10943, #2593, #19700, #312 ),
 .UNSPECIFIED., .F., .F.,
 ( 4, 2, 2, 2, 2, 2, 2, 4 ),
 ( 0.000000000000000000, 0.001557302553632665962, 0.002335953830448995582, 0.003114605107265324985, 0.004671907660898025859, 0.005450558937714371742, 0.005839884576122518663, 0.006229210214530665583 ),
 .UNSPECIFIED. ) ;
#22072=CARTESIAN_POINT ( 'NONE',  ( -274.7557459110829541, -165.0000000000001137, 86.12025961983464128 ) ) ;
#22097=AXIS2_PLACEMENT_3D ( 'NONE', #20324, #15746, #4802 ) ;
#22146=CARTESIAN_POINT ( 'NONE',  ( -210.0000000000000284, -157.0000000000000284, -105.0000000000000284 ) ) ;
#22150=CIRCLE ( 'NONE', #21701, 72.21503689626329958 ) ;
#22186=VERTEX_POINT ( 'NONE', #24188 ) ;
#22201=CARTESIAN_POINT ( 'NONE',  ( -268.0706223630187992, -170.6109535803436472, 94.24395792536559213 ) ) ;
#22219=VECTOR ( 'NONE', #15987, 1000.000000000000000 ) ;
#22223=VERTEX_POINT ( 'NONE', #9246 ) ;
#22225=DIRECTION ( 'NONE',  ( -0.4918581970360879074, 0.000000000000000000, 0.8706753206611571594 ) ) ;
#22239=AXIS2_PLACEMENT_3D ( 'NONE', #8835, #17029, #6115 ) ;
#22245=CYLINDRICAL_SURFACE ( 'NONE', #12120, 67.21503689626328537 ) ;
#22253=DIRECTION ( 'NONE',  ( 0.000000000000000000, 0.000000000000000000, -1.000000000000000000 ) ) ;
#22268=EDGE_CURVE ( 'NONE', #6741, #18918, #631, .T. ) ;
#22270=VERTEX_POINT ( 'NONE', #14270 ) ;
#22277=AXIS2_PLACEMENT_3D ( 'NONE', #13287, #28201, #26338 ) ;
#22344=EDGE_LOOP ( 'NONE', ( #14544, #4447, #12248, #3567 ) ) ;
#22378=DIRECTION ( 'NONE',  ( -1.000000000000000000, 0.000000000000000000, 0.000000000000000000 ) ) ;
#22398=ADVANCED_FACE ( 'NONE', ( #26015 ), #23589, .T. ) ;
#22400=DIRECTION ( 'NONE',  ( -0.000000000000000000, -1.000000000000000000, -0.000000000000000000 ) ) ;
#22458=ORIENTED_EDGE ( 'NONE', *, *, #5671, .T. ) ;
#22490=EDGE_CURVE ( 'NONE', #10018, #17075, #6336, .T. ) ;
#22518=CARTESIAN_POINT ( 'NONE',  ( -210.0000000000000568, -157.0000000000000284, -110.0000000000000284 ) ) ;
#22565=VERTEX_POINT ( 'NONE', #19840 ) ;
#22625=CARTESIAN_POINT ( 'NONE',  ( -260.0000000000001137, -165.0000000000001137, -59.99999999999986500 ) ) ;
#22635=EDGE_CURVE ( 'NONE', #6741, #17075, #22061, .T. ) ;
#22639=CARTESIAN_POINT ( 'NONE',  ( -275.9362193061379003, -170.0000000000001137, -102.1458326826622027 ) ) ;
#22644=ORIENTED_EDGE ( 'NONE', *, *, #11212, .T. ) ;
#22652=PLANE ( 'NONE',  #20450 ) ;
#22656=CARTESIAN_POINT ( 'NONE',  ( -276.0548825800837562, -164.9999999997509121, 107.4689643235781489 ) ) ;
#22747=DIRECTION ( 'NONE',  ( 0.000000000000000000, 0.000000000000000000, -1.000000000000000000 ) ) ;
#22748=DIRECTION ( 'NONE',  ( 4.540956701092242152E-16, 1.000000000000000000, 0.000000000000000000 ) ) ;
#22755=EDGE_CURVE ( 'NONE', #3702, #3368, #13028, .T. ) ;
#22757=CARTESIAN_POINT ( 'NONE',  ( -274.7557459110829541, -165.0000000000001137, -86.12025961983451339 ) ) ;
#22807=CYLINDRICAL_SURFACE ( 'NONE', #9785, 49.99999999999998579 ) ;
#22817=CARTESIAN_POINT ( 'NONE',  ( -210.0000000000000568, -152.0000000000000284, -105.0000000000000284 ) ) ;
#22841=CARTESIAN_POINT ( 'NONE',  ( -261.1919288306253293, -171.9377729149742038, -94.99999999999987210 ) ) ;
#22850=B_SPLINE_CURVE_WITH_KNOTS ( 'NONE', 3,
 ( #19575, #15556, #24305, #28311, #8659, #6496, #24033, #8793, #17552, #26315, #4611, #6640, #15419, #13400 ),
 .UNSPECIFIED., .F., .F.,
 ( 4, 2, 2, 2, 2, 2, 4 ),
 ( 0.000000000000000000, 0.001215459952587881953, 0.001823189928881842770, 0.002430919905175803804, 0.003038649881469764405, 0.003646379857763725439, 0.004861839810351617150 ),
 .UNSPECIFIED. ) ;
#22883=CIRCLE ( 'NONE', #3590, 5.000000000000004441 ) ;
#22944=DIRECTION ( 'NONE',  ( 0.000000000000000000, 0.000000000000000000, -1.000000000000000000 ) ) ;
#22947=EDGE_LOOP ( 'NONE', ( #19406, #23232, #5279, #14854 ) ) ;
#22958=DIRECTION ( 'NONE',  ( 0.000000000000000000, 0.000000000000000000, -1.000000000000000000 ) ) ;
#22976=DIRECTION ( 'NONE',  ( 0.000000000000000000, 0.000000000000000000, -1.000000000000000000 ) ) ;
#23018=DIRECTION ( 'NONE',  ( 2.775557561562887407E-16, 3.668437989309015850E-32, 1.000000000000000000 ) ) ;
#23019=ORIENTED_EDGE ( 'NONE', *, *, #27961, .T. ) ;
#23020=VECTOR ( 'NONE', #11397, 1000.000000000000000 ) ;
#23028=ADVANCED_FACE ( 'NONE', ( #13212 ), #22245, .F. ) ;
#23082=DIRECTION ( 'NONE',  ( 0.000000000000000000, 0.000000000000000000, 1.000000000000000000 ) ) ;
#23090=VERTEX_POINT ( 'NONE', #11488 ) ;
#23099=DIRECTION ( 'NONE',  ( -1.000000000000000000, 0.000000000000000000, 0.000000000000000000 ) ) ;
#23105=TOROIDAL_SURFACE ( 'NONE', #11661, 45.00000000000000711, 5.000000000000000000 ) ;
#23107=CARTESIAN_POINT ( 'NONE',  ( -266.0448161382843182, -170.9309335098052145, -94.61759932200439493 ) ) ;
#23150=VERTEX_POINT ( 'NONE', #26688 ) ;
#23159=CARTESIAN_POINT ( 'NONE',  ( -210.0000000000000853, -213.8933171992502196, -90.09368185681015007 ) ) ;
#23185=FACE_OUTER_BOUND ( 'NONE', #22947, .T. ) ;
#23213=CARTESIAN_POINT ( 'NONE',  ( -210.0000000000000568, -152.0000000000000284, 105.0000000000000284 ) ) ;
#23214=PLANE ( 'NONE',  #3345 ) ;
#23232=ORIENTED_EDGE ( 'NONE', *, *, #18603, .T. ) ;
#23245=CARTESIAN_POINT ( 'NONE',  ( -272.7483281375958200, -170.1453890489109142, 92.73246688958286654 ) ) ;
#23247=CARTESIAN_POINT ( 'NONE',  ( -261.1919288306253293, -171.9377729149742038, -104.9999999999998721 ) ) ;
#23265=ORIENTED_EDGE ( 'NONE', *, *, #10174, .F. ) ;
#23275=DIRECTION ( 'NONE',  ( 1.000000000000000000, 0.000000000000000000, 0.000000000000000000 ) ) ;
#23296=PLANE ( 'NONE',  #5377 ) ;
#23301=ORIENTED_EDGE ( 'NONE', *, *, #24046, .T. ) ;
#23307=DIRECTION ( 'NONE',  ( 1.000000000000000000, 0.000000000000000000, 2.775557561562887407E-16 ) ) ;
#23330=LINE ( 'NONE', #12430, #275 ) ;
#23334=CARTESIAN_POINT ( 'NONE',  ( -210.0000000000000568, -213.8933171992501627, -109.9063181431897789 ) ) ;
#23342=DIRECTION ( 'NONE',  ( 2.775557561562887407E-16, 3.668437989309015850E-32, -1.000000000000000000 ) ) ;
#23374=TOROIDAL_SURFACE ( 'NONE', #13297, 35.00000000000000711, 5.000000000000000000 ) ;
#23378=CARTESIAN_POINT ( 'NONE',  ( -270.0655465147688687, -165.1941129551596248, -88.29030773487120598 ) ) ;
#23434=FACE_OUTER_BOUND ( 'NONE', #11148, .T. ) ;
#23437=CARTESIAN_POINT ( 'NONE',  ( -290.0000000000001705, -220.0000000000000853, -59.99999999999987210 ) ) ;
#23471=CIRCLE ( 'NONE', #22097, 34.99999999999999289 ) ;
#23478=ORIENTED_EDGE ( 'NONE', *, *, #9846, .F. ) ;
#23519=CARTESIAN_POINT ( 'NONE',  ( -260.0000000000001137, -167.0819201924624906, -89.99999999999987210 ) ) ;
#23534=DIRECTION ( 'NONE',  ( -0.000000000000000000, -0.000000000000000000, 1.000000000000000000 ) ) ;
#23537=AXIS2_PLACEMENT_3D ( 'NONE', #24844, #26988, #24699 ) ;
#23545=VERTEX_POINT ( 'NONE', #9954 ) ;
#23565=ORIENTED_EDGE ( 'NONE', *, *, #20762, .F. ) ;
#23589=CYLINDRICAL_SURFACE ( 'NONE', #2410, 5.000000000000004441 ) ;
#23596=LINE ( 'NONE', #21432, #26052 ) ;
#23653=ORIENTED_EDGE ( 'NONE', *, *, #24445, .T. ) ;
#23666=CARTESIAN_POINT ( 'NONE',  ( -270.4051725677463764, -170.3149295705450186, -88.16521414542363289 ) ) ;
#23667=CARTESIAN_POINT ( 'NONE',  ( -261.2691008037259053, -166.7184843738689608, 90.00000000000001421 ) ) ;
#23705=DIRECTION ( 'NONE',  ( -3.053113317719176147E-15, -4.035281788239917819E-31, -1.000000000000000000 ) ) ;
#23718=EDGE_LOOP ( 'NONE', ( #25415, #16906, #26885, #28174 ) ) ;
#23754=ORIENTED_EDGE ( 'NONE', *, *, #22268, .F. ) ;
#23778=VECTOR ( 'NONE', #12600, 1000.000000000000000 ) ;
#23780=CARTESIAN_POINT ( 'NONE',  ( -272.4384950037861017, -165.0368469557824085, 87.33088399392040913 ) ) ;
#23787=AXIS2_PLACEMENT_3D ( 'NONE', #5820, #25366, #18756 ) ;
#23801=CARTESIAN_POINT ( 'NONE',  ( -211.9382648910248577, -218.8137564101509724, 92.60662834576568514 ) ) ;
#23847=CIRCLE ( 'NONE', #18801, 5.000000000000000888 ) ;
#23857=CARTESIAN_POINT ( 'NONE',  ( -277.2150368962633706, -170.0000000000001137, -101.5769467933888279 ) ) ;
#23868=AXIS2_PLACEMENT_3D ( 'NONE', #3577, #21252, #14379 ) ;
#23884=CARTESIAN_POINT ( 'NONE',  ( -277.2150368962633706, -170.0000000000001137, -101.5769467933888137 ) ) ;
#23896=CARTESIAN_POINT ( 'NONE',  ( -260.0000000000001137, -220.0000000000000853, -109.9999999999998721 ) ) ;
#23935=CARTESIAN_POINT ( 'NONE',  ( -261.1919288306253293, -171.9377729149742038, 95.00000000000004263 ) ) ;
#23943=CARTESIAN_POINT ( 'NONE',  ( -213.0248109774373688, -217.2055523511229467, 94.52687028321123819 ) ) ;
#23952=CARTESIAN_POINT ( 'NONE',  ( -274.7557459110828972, -170.0000000000001421, 86.12025961983464128 ) ) ;
#23975=ORIENTED_EDGE ( 'NONE', *, *, #27631, .T. ) ;
#24033=CARTESIAN_POINT ( 'NONE',  ( -211.7373893208448692, -220.0000000000001421, -107.1635277725268196 ) ) ;
#24046=EDGE_CURVE ( 'NONE', #19744, #13525, #8025, .T. ) ;
#24060=EDGE_CURVE ( 'NONE', #22186, #6357, #1292, .T. ) ;
#24078=CARTESIAN_POINT ( 'NONE',  ( -263.2465583119826533, -166.4129100889759059, 109.9213744122507990 ) ) ;
#24087=VECTOR ( 'NONE', #5881, 1000.000000000000000 ) ;
#24094=FACE_OUTER_BOUND ( 'NONE', #12565, .T. ) ;
#24097=EDGE_CURVE ( 'NONE', #28358, #17098, #11718, .T. ) ;
#24100=EDGE_CURVE ( 'NONE', #3224, #24757, #10725, .T. ) ;
#24103=DIRECTION ( 'NONE',  ( 0.000000000000000000, 0.000000000000000000, -1.000000000000000000 ) ) ;
#24188=CARTESIAN_POINT ( 'NONE',  ( -305.0000000000001137, -152.0000000000000284, -59.99999999999987210 ) ) ;
#24193=CARTESIAN_POINT ( 'NONE',  ( -261.1919288306253293, -171.9377729149742038, 105.0000000000000142 ) ) ;
#24194=CARTESIAN_POINT ( 'NONE',  ( -210.0000000000000568, -220.0000000000000853, -90.87829376371895762 ) ) ;
#24215=CARTESIAN_POINT ( 'NONE',  ( -262.5800650587033260, -171.5970377885955145, 95.00000000000000000 ) ) ;
#24222=CARTESIAN_POINT ( 'NONE',  ( -310.0000000000001137, -157.0000000000000284, -59.99999999999987210 ) ) ;
#24227=LINE ( 'NONE', #4261, #24554 ) ;
#24251=ORIENTED_EDGE ( 'NONE', *, *, #24100, .F. ) ;
#24292=CARTESIAN_POINT ( 'NONE',  ( -212.3316009019935962, -218.3936534609811133, 106.8607414965052556 ) ) ;
#24302=PLANE ( 'NONE',  #14334 ) ;
#24305=CARTESIAN_POINT ( 'NONE',  ( -212.1902760358752289, -220.0000000000001137, -105.8132860232897627 ) ) ;
#24331=ORIENTED_EDGE ( 'NONE', *, *, #5748, .T. ) ;
#24336=ORIENTED_EDGE ( 'NONE', *, *, #3407, .T. ) ;
#24346=CARTESIAN_POINT ( 'NONE',  ( -210.0000000000000568, -220.0000000000000853, 90.00000000000002842 ) ) ;
#24348=CARTESIAN_POINT ( 'NONE',  ( -275.9932544989950998, -170.0000000000001705, 91.21518331976510296 ) ) ;
#24365=CARTESIAN_POINT ( 'NONE',  ( -260.0000000000001137, -152.0000000000000284, 95.00000000000004263 ) ) ;
#24370=CARTESIAN_POINT ( 'NONE',  ( -260.0000000000001137, -157.0000000000000284, 60.00000000000002132 ) ) ;
#24380=ORIENTED_EDGE ( 'NONE', *, *, #25655, .T. ) ;
#24383=( LENGTH_UNIT ( ) NAMED_UNIT ( * ) SI_UNIT ( .MILLI., .METRE. ) );
#24385=ORIENTED_EDGE ( 'NONE', *, *, #25655, .F. ) ;
#24420=AXIS2_PLACEMENT_3D ( 'NONE', #10432, #1937, #5832 ) ;
#24423=VERTEX_POINT ( 'NONE', #23247 ) ;
#24445=EDGE_CURVE ( 'NONE', #10608, #6070, #17229, .T. ) ;
#24452=CARTESIAN_POINT ( 'NONE',  ( -260.0000000000001137, -165.0000000000001137, 60.00000000000002132 ) ) ;
#24500=ORIENTED_EDGE ( 'NONE', *, *, #9628, .F. ) ;
#24514=DIRECTION ( 'NONE',  ( -1.000000000000000000, -0.000000000000000000, -2.775557561562887407E-16 ) ) ;
#24523=ORIENTED_EDGE ( 'NONE', *, *, #13251, .F. ) ;
#24533=AXIS2_PLACEMENT_3D ( 'NONE', #4005, #10064, #23275 ) ;
#24536=EDGE_CURVE ( 'NONE', #28324, #23545, #19510, .T. ) ;
#24554=VECTOR ( 'NONE', #13323, 1000.000000000000000 ) ;
#24570=EDGE_CURVE ( 'NONE', #3147, #25123, #10795, .T. ) ;
#24674=AXIS2_PLACEMENT_3D ( 'NONE', #1329, #10240, #18998 ) ;
#24699=DIRECTION ( 'NONE',  ( 0.000000000000000000, 1.000000000000000000, 0.000000000000000000 ) ) ;
#24702=APPLICATION_CONTEXT ( 'automotive_design' ) ;
#24714=CIRCLE ( 'NONE', #23787, 30.00000000000002842 ) ;
#24744=AXIS2_PLACEMENT_3D ( 'NONE', #23437, #12820, #12683 ) ;
#24757=VERTEX_POINT ( 'NONE', #5555 ) ;
#24767=CARTESIAN_POINT ( 'NONE',  ( -264.4238960014317286, -166.0091389525178727, -89.67888693108041309 ) ) ;
#24803=CARTESIAN_POINT ( 'NONE',  ( -210.0000000000000568, -220.0000000000000853, 90.00000000000002842 ) ) ;
#24807=CARTESIAN_POINT ( 'NONE',  ( -261.6154359210910911, -166.7250444216647054, 110.0000000000000142 ) ) ;
#24815=CARTESIAN_POINT ( 'NONE',  ( -305.0000000000001137, -152.0000000000000284, 60.00000000000002842 ) ) ;
#24844=CARTESIAN_POINT ( 'NONE',  ( -210.0000000000000568, -157.0000000000000284, 95.00000000000004263 ) ) ;
#24898=ORIENTED_EDGE ( 'NONE', *, *, #19350, .F. ) ;
#24931=EDGE_CURVE ( 'NONE', #27204, #3702, #26130, .T. ) ;
#24932=DIRECTION ( 'NONE',  ( 1.000000000000000000, 1.321694076934710155E-16, -0.000000000000000000 ) ) ;
#24935=EDGE_CURVE ( 'NONE', #5617, #10903, #2830, .T. ) ;
#24953=CARTESIAN_POINT ( 'NONE',  ( -277.2150368962633706, -165.0000000000001421, 90.47363622314040299 ) ) ;
#24992=DIRECTION ( 'NONE',  ( 1.000000000000000000, -0.000000000000000000, 0.000000000000000000 ) ) ;
#25006=TOROIDAL_SURFACE ( 'NONE', #17676, 44.99999999999999289, 5.000000000000000000 ) ;
#25026=AXIS2_PLACEMENT_3D ( 'NONE', #13860, #22748, #9538 ) ;
#25029=AXIS2_PLACEMENT_3D ( 'NONE', #24370, #28376, #17200 ) ;
#25057=EDGE_CURVE ( 'NONE', #12396, #24423, #17531, .T. ) ;
#25065=CARTESIAN_POINT ( 'NONE',  ( 0.000000000000000000, 0.000000000000000000, 0.000000000000000000 ) ) ;
#25073=CARTESIAN_POINT ( 'NONE',  ( -210.0000000000000568, -157.0000000000000284, -94.99999999999987210 ) ) ;
#25077=VERTEX_POINT ( 'NONE', #2945 ) ;
#25097=ORIENTED_EDGE ( 'NONE', *, *, #21846, .T. ) ;
#25123=VERTEX_POINT ( 'NONE', #1212 ) ;
#25139=CYLINDRICAL_SURFACE ( 'NONE', #23868, 29.99999999999997158 ) ;
#25156=CARTESIAN_POINT ( 'NONE',  ( -260.0000000000001137, -167.0819201924624622, 95.00000000000002842 ) ) ;
#25165=EDGE_CURVE ( 'NONE', #2951, #22270, #23330, .T. ) ;
#25189=ORIENTED_EDGE ( 'NONE', *, *, #5032, .F. ) ;
#25192=CARTESIAN_POINT ( 'NONE',  ( -210.0000000000000568, -220.0000000000000853, 109.1217062362809145 ) ) ;
#25236=EDGE_LOOP ( 'NONE', ( #19232, #23565, #24500, #26569, #16070 ) ) ;
#25237=ORIENTED_EDGE ( 'NONE', *, *, #11489, .T. ) ;
#25281=FACE_OUTER_BOUND ( 'NONE', #14931, .T. ) ;
#25298=ORIENTED_EDGE ( 'NONE', *, *, #2472, .T. ) ;
#25320=CARTESIAN_POINT ( 'NONE',  ( -290.0000000000001137, -220.0000000000000853, 60.00000000000002842 ) ) ;
#25351=B_SPLINE_CURVE_WITH_KNOTS ( 'NONE', 3,
 ( #22757, #11845, #5499, #491, #9252, #9403, #16014, #20590, #24767, #5074, #13864, #17125 ),
 .UNSPECIFIED., .F., .F.,
 ( 4, 2, 2, 2, 2, 4 ),
 ( 0.000000000000000000, 0.003876131231190137454, 0.007752262462380274909, 0.009690328077975263188, 0.01162839369357025233, 0.01550452492476005022 ),
 .UNSPECIFIED. ) ;
#25365=CARTESIAN_POINT ( 'NONE',  ( -279.1278187736259611, -165.0000000000001421, 106.1966075482099541 ) ) ;
#25366=DIRECTION ( 'NONE',  ( -4.540956701092242152E-16, -1.000000000000000000, -0.000000000000000000 ) ) ;
#25379=CARTESIAN_POINT ( 'NONE',  ( -260.0000000000001137, -167.0819201924624622, -104.9999999999998721 ) ) ;
#25390=DIRECTION ( 'NONE',  ( 0.000000000000000000, 0.000000000000000000, 1.000000000000000000 ) ) ;
#25409=EDGE_CURVE ( 'NONE', #27440, #5806, #3457, .T. ) ;
#25415=ORIENTED_EDGE ( 'NONE', *, *, #7973, .T. ) ;
#25453=AXIS2_PLACEMENT_3D ( 'NONE', #8097, #19292, #26177 ) ;
#25458=CARTESIAN_POINT ( 'NONE',  ( -210.0000000000000568, -220.0000000000000853, 110.0000000000000284 ) ) ;
#25478=CARTESIAN_POINT ( 'NONE',  ( -277.2150368962633706, -237.2150368962634559, -104.9999999999998295 ) ) ;
#25522=ORIENTED_EDGE ( 'NONE', *, *, #16311, .T. ) ;
#25527=CARTESIAN_POINT ( 'NONE',  ( -211.8229433495291971, -220.0000000000000853, -93.01810040011434921 ) ) ;
#25567=CARTESIAN_POINT ( 'NONE',  ( -261.1919288306252724, -171.9377729149742038, -109.9999999999998721 ) ) ;
#25572=TOROIDAL_SURFACE ( 'NONE', #15990, 34.99999999999999289, 5.000000000000000000 ) ;
#25580=CARTESIAN_POINT ( 'NONE',  ( -208.4194785928031877, -215.2563777467642296, 60.00000000000002132 ) ) ;
#25617=CARTESIAN_POINT ( 'NONE',  ( -210.0000000000000853, -212.3568517473289887, -110.0000000000000568 ) ) ;
#25655=EDGE_CURVE ( 'NONE', #16800, #13530, #9932, .T. ) ;
#25667=CARTESIAN_POINT ( 'NONE',  ( -270.7973404499905428, -170.2932079548401987, -93.47773194822650566 ) ) ;
#25678=EDGE_LOOP ( 'NONE', ( #2073, #16886, #18809, #16240 ) ) ;
#25681=CARTESIAN_POINT ( 'NONE',  ( -277.2150368962633706, -170.0000000000001137, -110.0000000000000284 ) ) ;
#25748=VERTEX_POINT ( 'NONE', #17185 ) ;
#25750=EDGE_CURVE ( 'NONE', #17968, #25123, #25942, .T. ) ;
#25768=DIRECTION ( 'NONE',  ( 0.000000000000000000, 0.000000000000000000, -1.000000000000000000 ) ) ;
#25790=FACE_OUTER_BOUND ( 'NONE', #6550, .T. ) ;
#25806=CARTESIAN_POINT ( 'NONE',  ( -211.3305068427980586, -219.3267326664164614, 91.92140052019108509 ) ) ;
#25809=FACE_OUTER_BOUND ( 'NONE', #25678, .T. ) ;
#25811=CARTESIAN_POINT ( 'NONE',  ( -261.1919288306253293, -171.9377729149742038, 95.00000000000001421 ) ) ;
#25818=DIRECTION ( 'NONE',  ( 0.000000000000000000, 1.000000000000000000, 0.000000000000000000 ) ) ;
#25845=DIRECTION ( 'NONE',  ( 0.000000000000000000, 1.000000000000000000, 0.000000000000000000 ) ) ;
#25856=PRODUCT_DEFINITION_SHAPE ( 'NONE', 'NONE',  #3316 ) ;
#25893=CARTESIAN_POINT ( 'NONE',  ( -260.0000000000001137, -157.0000000000000284, -89.99999999999985789 ) ) ;
#25906=ORIENTED_EDGE ( 'NONE', *, *, #400, .F. ) ;
#25915=EDGE_CURVE ( 'NONE', #15321, #4251, #25996, .T. ) ;
#25942=LINE ( 'NONE', #865, #750 ) ;
#25954=CARTESIAN_POINT ( 'NONE',  ( -263.9486459716463855, -171.3073464501530907, -94.90637380402192491 ) ) ;
#25975=ORIENTED_EDGE ( 'NONE', *, *, #5223, .F. ) ;
#25996=CIRCLE ( 'NONE', #10860, 5.000000000000004441 ) ;
#25998=CARTESIAN_POINT ( 'NONE',  ( -271.7051148791218793, -170.2004882804717738, -108.6368843222754066 ) ) ;
#26006=ORIENTED_EDGE ( 'NONE', *, *, #11489, .F. ) ;
#26015=FACE_OUTER_BOUND ( 'NONE', #1732, .T. ) ;
#26052=VECTOR ( 'NONE', #10105, 1000.000000000000000 ) ;
#26056=CARTESIAN_POINT ( 'NONE',  ( -268.0136499788973765, -170.6190998804379717, 104.4234267195772219 ) ) ;
#26101=EDGE_CURVE ( 'NONE', #22270, #25748, #9305, .T. ) ;
#26115=AXIS2_PLACEMENT_3D ( 'NONE', #1411, #27964, #3699 ) ;
#26130=B_SPLINE_CURVE_WITH_KNOTS ( 'NONE', 3,
 ( #28223, #26491, #6823, #4519, #15180, #24078, #8566, #26217 ),
 .UNSPECIFIED., .F., .F.,
 ( 4, 2, 2, 4 ),
 ( 0.000000000000000000, 0.009823234264782376712, 0.01473485139717357027, 0.01964646852956476383 ),
 .UNSPECIFIED. ) ;
#26143=CARTESIAN_POINT ( 'NONE',  ( -275.9276330244907172, -170.0000000000001137, -102.1496523160547838 ) ) ;
#26156=FACE_OUTER_BOUND ( 'NONE', #12417, .T. ) ;
#26177=DIRECTION ( 'NONE',  ( 1.000000000000000000, 0.000000000000000000, 0.000000000000000000 ) ) ;
#26206=B_SPLINE_CURVE_WITH_KNOTS ( 'NONE', 3,
 ( #20520, #844, #7457, #16226, #21080, #14211 ),
 .UNSPECIFIED., .F., .F.,
 ( 4, 2, 4 ),
 ( 0.000000000000000000, 0.004615224477119856013, 0.009230448954239712026 ),
 .UNSPECIFIED. ) ;
#26213=ORIENTED_EDGE ( 'NONE', *, *, #20063, .T. ) ;
#26217=CARTESIAN_POINT ( 'NONE',  ( -260.0000000000001137, -167.0819201924624906, 110.0000000000000142 ) ) ;
#26251=ORIENTED_EDGE ( 'NONE', *, *, #2934, .F. ) ;
#26253=TOROIDAL_SURFACE ( 'NONE', #7899, 72.21503689626331379, 5.000000000000000000 ) ;
#26284=CARTESIAN_POINT ( 'NONE',  ( -260.0000000000001137, -170.0000000000001137, 60.00000000000002132 ) ) ;
#26312=VECTOR ( 'NONE', #17586, 1000.000000000000000 ) ;
#26315=CARTESIAN_POINT ( 'NONE',  ( -211.1960507716717643, -220.0000000000000568, -108.0220471272657363 ) ) ;
#26338=DIRECTION ( 'NONE',  ( 0.000000000000000000, 0.000000000000000000, 1.000000000000000000 ) ) ;
#26349=CARTESIAN_POINT ( 'NONE',  ( -270.0172489267828269, -165.2082603419176223, 88.28568317613442673 ) ) ;
#26357=CARTESIAN_POINT ( 'NONE',  ( -263.9606520309740176, -171.3050423792260801, 94.90504062136166397 ) ) ;
#26439=ORIENTED_EDGE ( 'NONE', *, *, #18193, .T. ) ;
#26489=LINE ( 'NONE', #24346, #7926 ) ;
#26491=CARTESIAN_POINT ( 'NONE',  ( -276.0611529335072305, -165.0000000000001137, 107.4663680683487001 ) ) ;
#26496=TOROIDAL_SURFACE ( 'NONE', #1727, 34.99999999999999289, 5.000000000000000000 ) ;
#26500=ORIENTED_EDGE ( 'NONE', *, *, #18595, .F. ) ;
#26507=DIRECTION ( 'NONE',  ( 4.540956701092242152E-16, 1.000000000000000000, 0.000000000000000000 ) ) ;
#26515=ORIENTED_EDGE ( 'NONE', *, *, #15464, .F. ) ;
#26539=ADVANCED_FACE ( 'NONE', ( #23434 ), #23296, .F. ) ;
#26555=DIRECTION ( 'NONE',  ( -1.000000000000000000, 4.540956701092242152E-16, 0.000000000000000000 ) ) ;
#26569=ORIENTED_EDGE ( 'NONE', *, *, #18603, .F. ) ;
#26589=DIRECTION ( 'NONE',  ( -1.000000000000000000, 0.000000000000000000, 3.053113317719176147E-15 ) ) ;
#26606=ORIENTED_EDGE ( 'NONE', *, *, #7973, .F. ) ;
#26647=ORIENTED_EDGE ( 'NONE', *, *, #1620, .T. ) ;
#26688=CARTESIAN_POINT ( 'NONE',  ( -310.0000000000001137, -157.0000000000000284, 60.00000000000002842 ) ) ;
#26713=ORIENTED_EDGE ( 'NONE', *, *, #21676, .F. ) ;
#26720=B_SPLINE_CURVE_WITH_KNOTS ( 'NONE', 3,
 ( #24193, #2064, #22034, #15579, #26056, #6666, #17865, #28200 ),
 .UNSPECIFIED., .F., .F.,
 ( 4, 2, 2, 4 ),
 ( 0.000000000000000000, 0.004191298939714996341, 0.008382597879429992682, 0.01676519575885998536 ),
 .UNSPECIFIED. ) ;
#26722=AXIS2_PLACEMENT_3D ( 'NONE', #9746, #23099, #25390 ) ;
#26732=EDGE_CURVE ( 'NONE', #5554, #23150, #15971, .T. ) ;
#26770=DIRECTION ( 'NONE',  ( -4.540956701092242152E-16, -1.000000000000000000, -0.000000000000000000 ) ) ;
#26874=DIRECTION ( 'NONE',  ( -1.321694076934710155E-16, 1.000000000000000000, 0.000000000000000000 ) ) ;
#26879=VECTOR ( 'NONE', #14691, 1000.000000000000000 ) ;
#26885=ORIENTED_EDGE ( 'NONE', *, *, #12010, .F. ) ;
#26937=ORIENTED_EDGE ( 'NONE', *, *, #17860, .F. ) ;
#26951=FACE_OUTER_BOUND ( 'NONE', #18491, .T. ) ;
#26988=DIRECTION ( 'NONE',  ( 1.000000000000000000, 1.321694076934710155E-16, 0.000000000000000000 ) ) ;
#26990=CARTESIAN_POINT ( 'NONE',  ( -260.0000000000001137, -167.0819201924624906, -89.99999999999985789 ) ) ;
#27062=DIRECTION ( 'NONE',  ( -1.000000000000000000, 5.551115123125784674E-16, 0.000000000000000000 ) ) ;
#27094=CARTESIAN_POINT ( 'NONE',  ( -273.2648702738334237, -170.0373740213163103, 108.3066405192712267 ) ) ;
#27111=ORIENTED_EDGE ( 'NONE', *, *, #26732, .F. ) ;
#27132=CARTESIAN_POINT ( 'NONE',  ( -290.0000000000001137, -165.0000000000000853, 60.00000000000002842 ) ) ;
#27138=CARTESIAN_POINT ( 'NONE',  ( -260.0000000000001137, -157.0000000000000284, -104.9999999999998721 ) ) ;
#27149=CARTESIAN_POINT ( 'NONE',  ( -310.0000000000001137, -220.0000000000000853, 60.00000000000002842 ) ) ;
#27163=LINE ( 'NONE', #25681, #22219 ) ;
#27181=CARTESIAN_POINT ( 'NONE',  ( -210.0000000000000000, -212.3568517473289035, -89.99999999999990052 ) ) ;
#27204=VERTEX_POINT ( 'NONE', #8888 ) ;
#27206=CARTESIAN_POINT ( 'NONE',  ( -210.0000000000000568, -220.0000000000000853, -110.0000000000000284 ) ) ;
#27214=VECTOR ( 'NONE', #22747, 1000.000000000000000 ) ;
#27270=VERTEX_POINT ( 'NONE', #5564 ) ;
#27276=ORIENTED_EDGE ( 'NONE', *, *, #9846, .T. ) ;
#27309=ORIENTED_EDGE ( 'NONE', *, *, #24046, .F. ) ;
#27316=DIRECTION ( 'NONE',  ( -1.000000000000000000, 0.000000000000000000, 0.000000000000000000 ) ) ;
#27329=CARTESIAN_POINT ( 'NONE',  ( -210.0000000000000568, -152.0000000000000284, -94.99999999999987210 ) ) ;
#27338=CARTESIAN_POINT ( 'NONE',  ( -260.0000000000001137, -157.0000000000000284, -59.99999999999986500 ) ) ;
#27373=EDGE_LOOP ( 'NONE', ( #17134, #26439, #8282, #25237, #12158 ) ) ;
#27378=ORIENTED_EDGE ( 'NONE', *, *, #6567, .T. ) ;
#27387=CARTESIAN_POINT ( 'NONE',  ( -211.1943141956539876, -220.0000000000000853, -91.97569866068964473 ) ) ;
#27436=DIRECTION ( 'NONE',  ( -0.9711705445023439687, 0.2383857661250367854, 0.000000000000000000 ) ) ;
#27440=VERTEX_POINT ( 'NONE', #6555 ) ;
#27479=CIRCLE ( 'NONE', #14655, 50.00000000000000711 ) ;
#27505=CARTESIAN_POINT ( 'NONE',  ( -263.2377953986417651, -166.4145296663307647, 109.9218949472355291 ) ) ;
#27541=DIRECTION ( 'NONE',  ( -0.9239321509641975627, -1.061807240666849658E-15, 0.3825563754725197496 ) ) ;
#27554=ORIENTED_EDGE ( 'NONE', *, *, #27847, .F. ) ;
#27561=EDGE_CURVE ( 'NONE', #268, #301, #27479, .T. ) ;
#27565=ADVANCED_FACE ( 'NONE', ( #13998 ), #1041, .F. ) ;
#27570=CARTESIAN_POINT ( 'NONE',  ( -277.2150368962633706, -237.2150368962634559, -94.99999999999985789 ) ) ;
#27592=ORIENTED_EDGE ( 'NONE', *, *, #16469, .F. ) ;
#27605=EDGE_CURVE ( 'NONE', #21916, #10608, #17851, .T. ) ;
#27631=EDGE_CURVE ( 'NONE', #27204, #25077, #10512, .T. ) ;
#27637=LINE ( 'NONE', #16601, #16299 ) ;
#27661=EDGE_LOOP ( 'NONE', ( #5382, #16127, #5662, #22011, #21036, #13698 ) ) ;
#27671=CARTESIAN_POINT ( 'NONE',  ( -273.6827204801242601, -170.0454132223111969, -86.72642857975071706 ) ) ;
#27673=CARTESIAN_POINT ( 'NONE',  ( -274.7077367163463464, -170.0340389212390448, 91.88143064332926713 ) ) ;
#27712=DIRECTION ( 'NONE',  ( 2.775557561562887407E-16, 3.668437989309015850E-32, 1.000000000000000000 ) ) ;
#27718=FACE_OUTER_BOUND ( 'NONE', #9348, .T. ) ;
#27724=CARTESIAN_POINT ( 'NONE',  ( -260.0000000000001137, -165.0000000000000853, 60.00000000000002132 ) ) ;
#27732=MANIFOLD_SOLID_BREP ( 'Fillet9', #20051 ) ;
#27734=CYLINDRICAL_SURFACE ( 'NONE', #6373, 5.000000000000004441 ) ;
#27738=AXIS2_PLACEMENT_3D ( 'NONE', #17450, #5969, #15318 ) ;
#27739=CARTESIAN_POINT ( 'NONE',  ( -213.1827219047386848, -216.7767438708612531, -110.0000000000000284 ) ) ;
#27748=CIRCLE ( 'NONE', #2992, 44.99999999999998579 ) ;
#27757=DIRECTION ( 'NONE',  ( 4.625929269271489858E-16, -2.100614451407711032E-31, 1.000000000000000000 ) ) ;
#27760=DIRECTION ( 'NONE',  ( -3.053113317719176147E-15, -4.035281788239917819E-31, -1.000000000000000000 ) ) ;
#27778=LINE ( 'NONE', #10411, #710 ) ;
#27806=ORIENTED_EDGE ( 'NONE', *, *, #17610, .F. ) ;
#27809=CARTESIAN_POINT ( 'NONE',  ( -210.0000000000000568, -220.0000000000000853, 90.87829376371914236 ) ) ;
#27828=ORIENTED_EDGE ( 'NONE', *, *, #6135, .F. ) ;
#27842=CARTESIAN_POINT ( 'NONE',  ( -305.0000000000001137, -152.0000000000000284, 60.00000000000001421 ) ) ;
#27847=EDGE_CURVE ( 'NONE', #23150, #268, #16352, .T. ) ;
#27879=EDGE_CURVE ( 'NONE', #23150, #6357, #21475, .T. ) ;
#27894=CARTESIAN_POINT ( 'NONE',  ( -210.0000000000000568, -157.0000000000000284, 110.0000000000000284 ) ) ;
#27951=CARTESIAN_POINT ( 'NONE',  ( -274.7557459110829541, -165.0000000000001137, -86.12025961983451339 ) ) ;
#27961=EDGE_CURVE ( 'NONE', #21738, #22565, #6116, .T. ) ;
#27964=DIRECTION ( 'NONE',  ( 0.000000000000000000, 1.000000000000000000, 0.000000000000000000 ) ) ;
#27973=ORIENTED_EDGE ( 'NONE', *, *, #25915, .F. ) ;
#28010=ADVANCED_FACE ( 'NONE', ( #10008 ), #7990, .T. ) ;
#28021=CARTESIAN_POINT ( 'NONE',  ( -210.0000000000000568, -220.0000000000000853, -110.0000000000000284 ) ) ;
#28050=EDGE_CURVE ( 'NONE', #6070, #13530, #4658, .T. ) ;
#28096=CARTESIAN_POINT ( 'NONE',  ( -263.5400929610141247, -171.3942524661753453, -89.83009453516376652 ) ) ;
#28097=CARTESIAN_POINT ( 'NONE',  ( -260.0000000000001137, -167.0819201924624906, 90.00000000000001421 ) ) ;
#28100=CARTESIAN_POINT ( 'NONE',  ( -268.1197270641252430, -170.6145491720722589, -94.20778360409461527 ) ) ;
#28133=FACE_OUTER_BOUND ( 'NONE', #17118, .T. ) ;
#28137=DIRECTION ( 'NONE',  ( 0.000000000000000000, 0.000000000000000000, -1.000000000000000000 ) ) ;
#28145=CARTESIAN_POINT ( 'NONE',  ( -266.5933816631180662, -170.7896271858165278, -104.7207418755312744 ) ) ;
#28174=ORIENTED_EDGE ( 'NONE', *, *, #22027, .T. ) ;
#28200=CARTESIAN_POINT ( 'NONE',  ( -277.2150368962633706, -170.0000000000001137, 101.5769467933889558 ) ) ;
#28201=DIRECTION ( 'NONE',  ( -1.000000000000000000, 0.000000000000000000, 0.000000000000000000 ) ) ;
#28205=EDGE_CURVE ( 'NONE', #23090, #8779, #23471, .T. ) ;
#28221=DIRECTION ( 'NONE',  ( 1.000000000000000000, 1.321694076934710155E-16, -0.000000000000000000 ) ) ;
#28223=CARTESIAN_POINT ( 'NONE',  ( -279.1278187736259611, -165.0000000000001421, 106.1966075482099399 ) ) ;
#28233=FACE_OUTER_BOUND ( 'NONE', #4284, .T. ) ;
#28237=CARTESIAN_POINT ( 'NONE',  ( -261.2693309676747617, -166.7184184611137709, -89.99999999999987210 ) ) ;
#28239=CARTESIAN_POINT ( 'NONE',  ( -268.1741054074460635, -165.4056554755341892, 88.87211405343852277 ) ) ;
#28274=CARTESIAN_POINT ( 'NONE',  ( -277.2150368962633706, -237.2150368962634559, -110.0000000000000284 ) ) ;
#28277=DIRECTION ( 'NONE',  ( 0.000000000000000000, 0.000000000000000000, -1.000000000000000000 ) ) ;
#28279=DIRECTION ( 'NONE',  ( -1.000000000000000000, 6.167905692361982533E-16, 1.850371707708594760E-15 ) ) ;
#28286=CARTESIAN_POINT ( 'NONE',  ( -263.8977010603396138, -171.2736078107176638, -104.9999999999167812 ) ) ;
#28289=VERTEX_POINT ( 'NONE', #16169 ) ;
#28301=CARTESIAN_POINT ( 'NONE',  ( -212.9132412317957233, -217.4562798785298128, 105.7556772048274922 ) ) ;
#28311=CARTESIAN_POINT ( 'NONE',  ( -212.0383327733632370, -220.0000000000000284, -106.4038250379320516 ) ) ;
#28324=VERTEX_POINT ( 'NONE', #5936 ) ;
#28358=VERTEX_POINT ( 'NONE', #7958 ) ;
#28364=CARTESIAN_POINT ( 'NONE',  ( -212.9132412317957233, -217.4562798785298128, 94.24432279517255040 ) ) ;
#28376=DIRECTION ( 'NONE',  ( 0.000000000000000000, 1.000000000000000000, 0.000000000000000000 ) ) ;
#28386=VECTOR ( 'NONE', #13434, 1000.000000000000000 ) ;
#28393=AXIS2_PLACEMENT_3D ( 'NONE', #15491, #8730, #17206 ) ;
#28414=COLOUR_RGB('Dark Blue',0.08,0.2,0.34);
#28415=FILL_AREA_STYLE_COLOUR('',#28414);
#28416=FILL_AREA_STYLE('',(#28415));
#28417=SURFACE_STYLE_FILL_AREA(#28416);
#28418=SURFACE_SIDE_STYLE('',(#28417));
#28419=SURFACE_STYLE_USAGE(.BOTH.,#28418);
#28420=PRESENTATION_STYLE_ASSIGNMENT((#28419));
ENDSEC;
END-ISO-10303-21;
